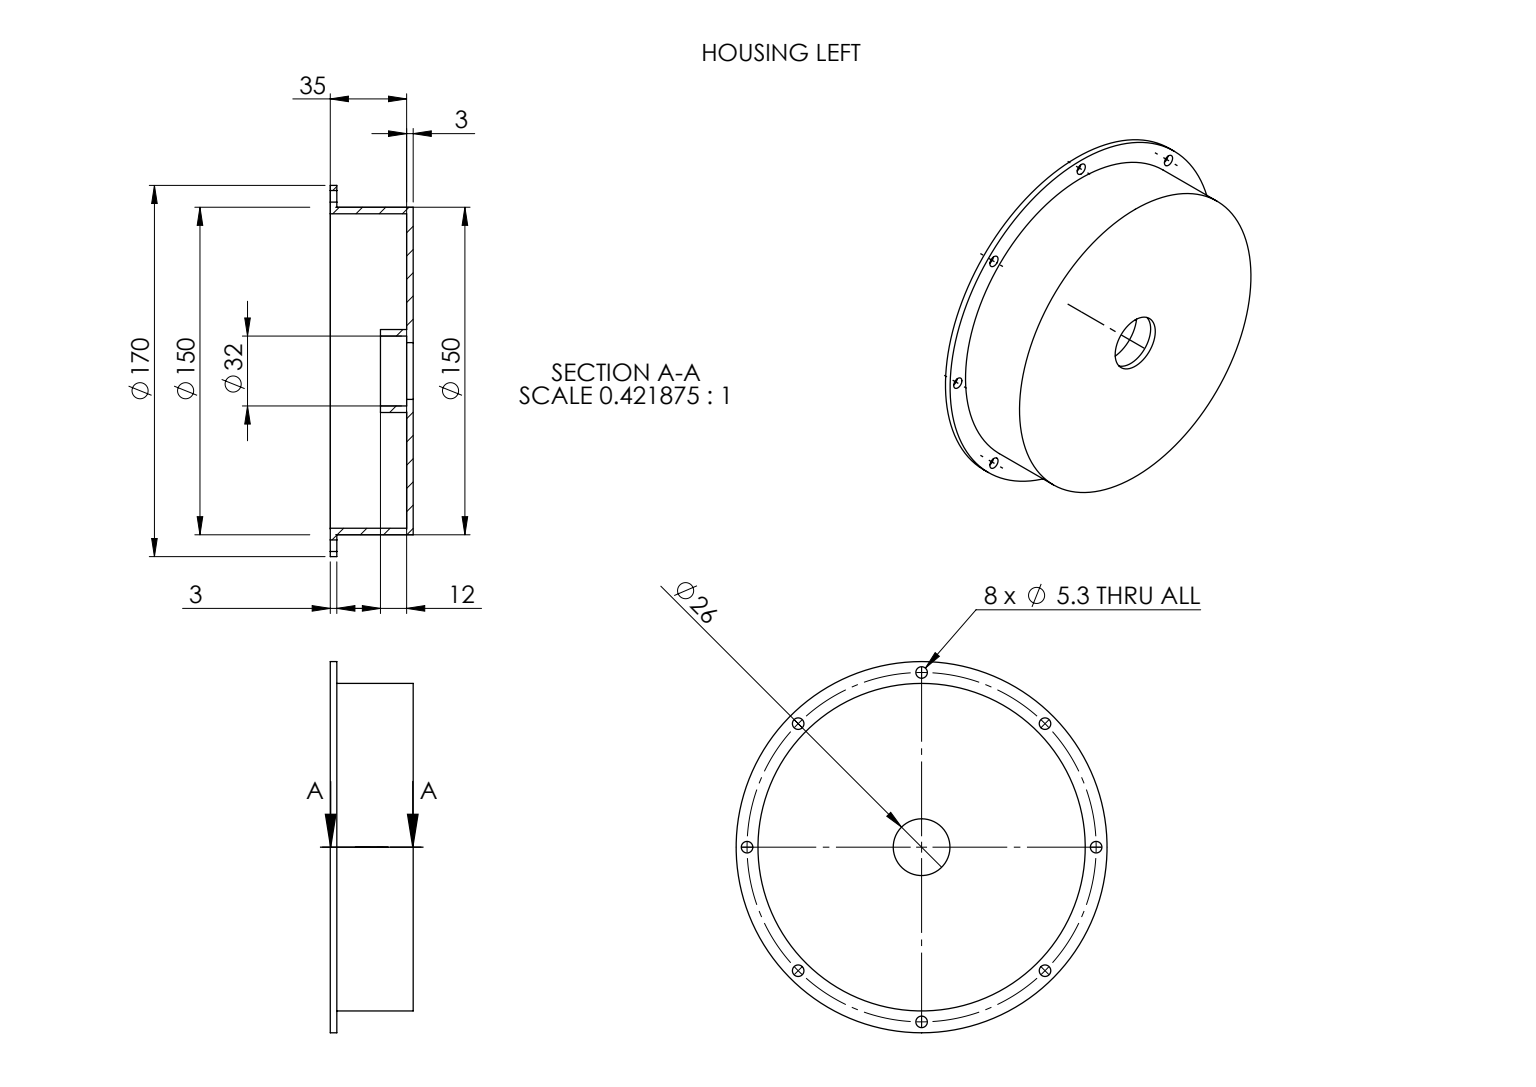
ISO-10303-21;
HEADER;
FILE_DESCRIPTION (('STEP AP214'),
    '1' );
FILE_NAME ('housing left.step',
    '2026-10-08T08:02:49',
    ( '' ),
    ( '' ),
    'SwSTEP 2.0',
    'SolidWorks 2026',
    '' );
FILE_SCHEMA (( 'AUTOMOTIVE_DESIGN' ));
ENDSEC;

DATA;
#22=CIRCLE ( 'NONE', #14059, 18.99999999999999645 ) ;
#26=ORIENTED_EDGE ( 'NONE', *, *, #59034, .F. ) ;
#28=CARTESIAN_POINT ( 'NONE',  ( 9.999999999999994671, 54.69470952477936976, 58.44237546506825964 ) ) ;
#114=DIRECTION ( 'NONE',  ( 0.000000000000000000, 0.7071067811865540120, -0.7071067811865409114 ) ) ;
#229=DIRECTION ( 'NONE',  ( -1.558861125776144859E-16, 1.000000000000000000, 0.000000000000000000 ) ) ;
#516=VERTEX_POINT ( 'NONE', #28669 ) ;
#583=FILL_AREA_STYLE_COLOUR ( '', #10848 ) ;
#732=EDGE_CURVE ( 'NONE', #32675, #50174, #22, .T. ) ;
#739=EDGE_LOOP ( 'NONE', ( #30578, #30226 ) ) ;
#851=EDGE_CURVE ( 'NONE', #38431, #10608, #42121, .T. ) ;
#979=CARTESIAN_POINT ( 'NONE',  ( 7.000000000000016875, -56.56854249492410958, 56.56854249492351983 ) ) ;
#1004=DIRECTION ( 'NONE',  ( 0.000000000000000000, 0.7071067811865500152, -0.7071067811865449082 ) ) ;
#1045=EDGE_CURVE ( 'NONE', #44352, #37554, #11099, .T. ) ;
#1056=AXIS2_PLACEMENT_3D ( 'NONE', #46617, #46933, #37219 ) ;
#1220=EDGE_LOOP ( 'NONE', ( #16192, #58248 ) ) ;
#1238=FACE_OUTER_BOUND ( 'NONE', #25127, .T. ) ;
#1308=ADVANCED_FACE ( 'NONE', ( #34786, #1238 ), #48554, .F. ) ;
#1325=EDGE_CURVE ( 'NONE', #18038, #2711, #15080, .T. ) ;
#1357=VERTEX_POINT ( 'NONE', #29143 ) ;
#1407=MECHANICAL_DESIGN_GEOMETRIC_PRESENTATION_REPRESENTATION('',(#54392),#17442);
#1450=EDGE_CURVE ( 'NONE', #1988, #10608, #40149, .T. ) ;
#1480=ORIENTED_EDGE ( 'NONE', *, *, #24999, .F. ) ;
#1544=ORIENTED_EDGE ( 'NONE', *, *, #24999, .T. ) ;
#1597=PRODUCT_DEFINITION_CONTEXT ( 'detailed design', #21992, 'design' ) ;
#1693=EDGE_LOOP ( 'NONE', ( #9790, #42814, #6756, #22247 ) ) ;
#1722=LINE ( 'NONE', #34653, #61604 ) ;
#1747=FACE_BOUND ( 'NONE', #39086, .T. ) ;
#1845=ORIENTED_EDGE ( 'NONE', *, *, #29444, .T. ) ;
#1874=VERTEX_POINT ( 'NONE', #54743 ) ;
#1982=VECTOR ( 'NONE', #50943, 1000.000000000000000 ) ;
#1983=FACE_BOUND ( 'NONE', #59580, .T. ) ;
#1988=VERTEX_POINT ( 'NONE', #18412 ) ;
#2034=ADVANCED_FACE ( 'NONE', ( #24026, #4272 ), #4895, .F. ) ;
#2113=DIRECTION ( 'NONE',  ( -1.000000000000000000, -1.836909530733573776E-16, 1.925929944387235853E-32 ) ) ;
#2157=EDGE_CURVE ( 'NONE', #55402, #25319, #24135, .T. ) ;
#2440=AXIS2_PLACEMENT_3D ( 'NONE', #41505, #59968, #8898 ) ;
#2557=DIRECTION ( 'NONE',  ( 0.000000000000000000, -1.000000000000000000, 0.000000000000000000 ) ) ;
#2571=CARTESIAN_POINT ( 'NONE',  ( 7.000000000000006217, 8.392413579938656024E-13, -80.00000000000001421 ) ) ;
#2625=EDGE_LOOP ( 'NONE', ( #36396, #26501, #31258, #19273 ) ) ;
#2659=AXIS2_PLACEMENT_3D ( 'NONE', #51775, #8874, #36245 ) ;
#2684=DIRECTION ( 'NONE',  ( -1.000000000000000000, -0.000000000000000000, -0.000000000000000000 ) ) ;
#2711=VERTEX_POINT ( 'NONE', #24485 ) ;
#2720=CIRCLE ( 'NONE', #37781, 2.649999999999999467 ) ;
#2736=ORIENTED_EDGE ( 'NONE', *, *, #34296, .T. ) ;
#2739=LINE ( 'NONE', #12480, #41873 ) ;
#2753=CIRCLE ( 'NONE', #37812, 2.649999999999985700 ) ;
#2770=CYLINDRICAL_SURFACE ( 'NONE', #48946, 2.649999999999992806 ) ;
#2778=DIRECTION ( 'NONE',  ( -1.000000000000000000, -1.836909530733573776E-16, 1.103352205049209901E-32 ) ) ;
#2817=MECHANICAL_DESIGN_GEOMETRIC_PRESENTATION_REPRESENTATION('',(#48840),#50847);
#2821=EDGE_CURVE ( 'NONE', #57549, #39665, #59140, .T. ) ;
#2917=EDGE_CURVE ( 'NONE', #47400, #1357, #48167, .T. ) ;
#3017=VERTEX_POINT ( 'NONE', #18490 ) ;
#3042=CARTESIAN_POINT ( 'NONE',  ( 42.00000000000000711, 6.547216728259810428E-15, -1.617781153285278467E-30 ) ) ;
#3179=EDGE_LOOP ( 'NONE', ( #47636, #54086, #41638, #28463 ) ) ;
#3190=CARTESIAN_POINT ( 'NONE',  ( 10.00000000000000533, 8.397924308530857731E-13, -80.00000000000001421 ) ) ;
#3221=DIRECTION ( 'NONE',  ( -1.000000000000000000, -0.000000000000000000, -0.000000000000000000 ) ) ;
#3238=ORIENTED_EDGE ( 'NONE', *, *, #53930, .F. ) ;
#3304=CARTESIAN_POINT ( 'NONE',  ( 42.00000000000000711, 7.715020029081011437E-15, -8.088905766426392334E-31 ) ) ;
#3387=VERTEX_POINT ( 'NONE', #31748 ) ;
#3408=ADVANCED_FACE ( 'NONE', ( #35844, #26731, #45253, #16411, #44942, #55220, #12654, #54282, #1983, #21108 ), #11405, .T. ) ;
#3479=VERTEX_POINT ( 'NONE', #8534 ) ;
#3488=DIRECTION ( 'NONE',  ( 1.000000000000000000, 1.836909530733573776E-16, -1.925929944387235579E-32 ) ) ;
#3501=DIRECTION ( 'NONE',  ( -1.000000000000000000, -5.380183451256670742E-17, 1.298891185607911324E-16 ) ) ;
#3546=CIRCLE ( 'NONE', #38604, 72.00000000000002842 ) ;
#3620=CARTESIAN_POINT ( 'NONE',  ( 7.000000000000016875, -54.69470952477895054, -58.44237546506863623 ) ) ;
#3624=CARTESIAN_POINT ( 'NONE',  ( 30.00000000000000711, 19.00000000000000000, -1.386669559958810165E-30 ) ) ;
#3759=CARTESIAN_POINT ( 'NONE',  ( 0.000000000000000000, 0.000000000000000000, 0.000000000000000000 ) ) ;
#3767=VECTOR ( 'NONE', #5831, 1000.000000000000000 ) ;
#3775=PRODUCT ( 'housing left', 'housing left', '', ( #26178 ) ) ;
#3842=DIRECTION ( 'NONE',  ( -1.000000000000000000, -3.135800716341471541E-16, -1.298891185607920445E-16 ) ) ;
#3848=CARTESIAN_POINT ( 'NONE',  ( 30.00000000000001066, 4.342925291379521108E-15, -1.386669559958810165E-30 ) ) ;
#3874=CARTESIAN_POINT ( 'NONE',  ( 7.000000000000021316, -80.00000000000001421, 2.649999999999992806 ) ) ;
#4007=VERTEX_POINT ( 'NONE', #26972 ) ;
#4020=EDGE_CURVE ( 'NONE', #3387, #24101, #40936, .T. ) ;
#4024=EDGE_LOOP ( 'NONE', ( #28100, #44874 ) ) ;
#4063=ORIENTED_EDGE ( 'NONE', *, *, #5152, .T. ) ;
#4173=DIRECTION ( 'NONE',  ( -1.000000000000000000, -1.836909530733573776E-16, 1.925929944387234758E-32 ) ) ;
#4221=ADVANCED_FACE ( 'NONE', ( #22092 ), #31172, .F. ) ;
#4236=EDGE_LOOP ( 'NONE', ( #11283, #12412 ) ) ;
#4258=CARTESIAN_POINT ( 'NONE',  ( 10.00000000000000533, 2.650000000000832134, -79.99999999999998579 ) ) ;
#4272=FACE_OUTER_BOUND ( 'NONE', #21523, .T. ) ;
#4292=DIRECTION ( 'NONE',  ( -1.826024711554534160E-16, 1.000000000000000000, 0.000000000000000000 ) ) ;
#4309=EDGE_CURVE ( 'NONE', #25319, #44352, #60010, .T. ) ;
#4456=AXIS2_PLACEMENT_3D ( 'NONE', #52364, #46164, #18264 ) ;
#4472=AXIS2_PLACEMENT_3D ( 'NONE', #56348, #47281, #33193 ) ;
#4491=CYLINDRICAL_SURFACE ( 'NONE', #43043, 15.99999999999999645 ) ;
#4503=CARTESIAN_POINT ( 'NONE',  ( 10.00000000000000888, -2.549224068967256091E-30, 75.00000000000001421 ) ) ;
#4529=AXIS2_PLACEMENT_3D ( 'NONE', #47141, #35361, #8584 ) ;
#4613=ORIENTED_EDGE ( 'NONE', *, *, #10966, .T. ) ;
#4647=ORIENTED_EDGE ( 'NONE', *, *, #16498, .T. ) ;
#4759=DIRECTION ( 'NONE',  ( -1.000000000000000000, -3.673819061467147552E-16, 1.925929944387234758E-32 ) ) ;
#4811=DIRECTION ( 'NONE',  ( -1.000000000000000000, -3.135800716341471541E-16, -1.298891185607920445E-16 ) ) ;
#4817=DIRECTION ( 'NONE',  ( 0.000000000000000000, 0.000000000000000000, 1.000000000000000000 ) ) ;
#4831=ADVANCED_BREP_SHAPE_REPRESENTATION ( '', ( #52245, #14677 ), #24835 ) ;
#4895=PLANE ( 'NONE',  #1056 ) ;
#4898=DIRECTION ( 'NONE',  ( 3.273063162220391312E-16, -1.000000000000000000, -5.236901059552626099E-15 ) ) ;
#4917=ORIENTED_EDGE ( 'NONE', *, *, #7261, .F. ) ;
#5152=EDGE_CURVE ( 'NONE', #20064, #24696, #61930, .T. ) ;
#5167=ORIENTED_EDGE ( 'NONE', *, *, #2821, .F. ) ;
#5171=LINE ( 'NONE', #6084, #41199 ) ;
#5227=ADVANCED_FACE ( 'NONE', ( #32227 ), #2770, .F. ) ;
#5259=EDGE_LOOP ( 'NONE', ( #10232, #39171, #52640, #43675 ) ) ;
#5271=CARTESIAN_POINT ( 'NONE',  ( 6.999999999999995559, 58.44237546506807490, 54.69470952477956871 ) ) ;
#5291=DIRECTION ( 'NONE',  ( -1.000000000000000000, -5.380183451256670742E-17, 1.298891185607911324E-16 ) ) ;
#5452=ORIENTED_EDGE ( 'NONE', *, *, #1325, .T. ) ;
#5519=FACE_BOUND ( 'NONE', #54215, .T. ) ;
#5603=ORIENTED_EDGE ( 'NONE', *, *, #43200, .F. ) ;
#5607=DIRECTION ( 'NONE',  ( -1.000000000000000000, -3.135800716341489291E-16, 1.298891185607901956E-16 ) ) ;
#5609=ORIENTED_EDGE ( 'NONE', *, *, #29444, .F. ) ;
#5821=DIRECTION ( 'NONE',  ( 1.836909530733573776E-16, -1.000000000000000000, 0.000000000000000000 ) ) ;
#5831=DIRECTION ( 'NONE',  ( -1.000000000000000000, -0.000000000000000000, -0.000000000000000000 ) ) ;
#5915=EDGE_LOOP ( 'NONE', ( #46556, #34430, #13398, #58645 ) ) ;
#6084=CARTESIAN_POINT ( 'NONE',  ( 6.999999999999992895, 72.00000000000002842, -1.348150961071066192E-31 ) ) ;
#6112=CARTESIAN_POINT ( 'NONE',  ( 30.00000000000000711, 16.00000000000000000, -1.502225356622044316E-30 ) ) ;
#6135=AXIS2_PLACEMENT_3D ( 'NONE', #35539, #54601, #49302 ) ;
#6151=CARTESIAN_POINT ( 'NONE',  ( 6.999999999999995559, 56.56854249492450037, -56.56854249492312192 ) ) ;
#6161=EDGE_CURVE ( 'NONE', #33929, #20064, #41040, .T. ) ;
#6225=DIRECTION ( 'NONE',  ( -1.000000000000000000, -3.135800716341471541E-16, -1.298891185607920445E-16 ) ) ;
#6490=VECTOR ( 'NONE', #52929, 1000.000000000000000 ) ;
#6576=CARTESIAN_POINT ( 'NONE',  ( 10.00000000000001599, -56.56854249492331377, -56.56854249492430142 ) ) ;
#6600=ORIENTED_EDGE ( 'NONE', *, *, #12325, .T. ) ;
#6625=DIRECTION ( 'NONE',  ( -3.273063162220391312E-16, 1.000000000000000000, 1.047380211910525220E-14 ) ) ;
#6709=DIRECTION ( 'NONE',  ( 1.836766033387207149E-16, -1.000000000000000000, 0.000000000000000000 ) ) ;
#6756=ORIENTED_EDGE ( 'NONE', *, *, #44992, .T. ) ;
#6760=SHAPE_REPRESENTATION ( 'housing left', ( #14677 ), #24835 ) ;
#6863=AXIS2_PLACEMENT_3D ( 'NONE', #23333, #47761, #37770 ) ;
#7077=CARTESIAN_POINT ( 'NONE',  ( 42.00000000000000711, 1.592040838891559293E-15, -13.00000000000000178 ) ) ;
#7123=FACE_BOUND ( 'NONE', #19230, .T. ) ;
#7125=CIRCLE ( 'NONE', #18162, 2.649999999999997691 ) ;
#7151=LINE ( 'NONE', #12514, #53981 ) ;
#7225=CARTESIAN_POINT ( 'NONE',  ( 45.00000000000001421, 0.000000000000000000, 0.000000000000000000 ) ) ;
#7261=EDGE_CURVE ( 'NONE', #50174, #32675, #28553, .T. ) ;
#7264=CARTESIAN_POINT ( 'NONE',  ( 9.999999999999991118, 80.00000000000001421, 2.649999999999992806 ) ) ;
#7288=CARTESIAN_POINT ( 'NONE',  ( 7.000000000000006217, 1.285836671513502038E-15, -1.348150961071066192E-31 ) ) ;
#7300=CYLINDRICAL_SURFACE ( 'NONE', #35562, 18.99999999999999645 ) ;
#7334=EDGE_CURVE ( 'NONE', #43245, #53393, #46557, .T. ) ;
#7452=ORIENTED_EDGE ( 'NONE', *, *, #34318, .F. ) ;
#7487=EDGE_LOOP ( 'NONE', ( #36785, #12533, #57073, #23756 ) ) ;
#7625=DIRECTION ( 'NONE',  ( 0.000000000000000000, 0.000000000000000000, 1.000000000000000000 ) ) ;
#7658=VECTOR ( 'NONE', #27391, 1000.000000000000000 ) ;
#7679=EDGE_LOOP ( 'NONE', ( #1480, #38792, #47540, #22144 ) ) ;
#7754=DIRECTION ( 'NONE',  ( -1.000000000000000000, -1.836909530733573776E-16, 1.925929944387235853E-32 ) ) ;
#7877=PRODUCT_DEFINITION_FORMATION_WITH_SPECIFIED_SOURCE ( 'ANY', '', #3775, .NOT_KNOWN. ) ;
#7972=LINE ( 'NONE', #3874, #59630 ) ;
#7976=FACE_OUTER_BOUND ( 'NONE', #29688, .T. ) ;
#8009=DIRECTION ( 'NONE',  ( 0.000000000000000000, -1.047444401652941269E-14, 1.000000000000000000 ) ) ;
#8045=DIRECTION ( 'NONE',  ( -1.000000000000000000, -5.380183451256491399E-17, -1.298891185607892835E-16 ) ) ;
#8080=DIRECTION ( 'NONE',  ( -1.000000000000000000, -1.836909530733573776E-16, 1.925929944387235853E-32 ) ) ;
#8132=CYLINDRICAL_SURFACE ( 'NONE', #55782, 2.649999999999992806 ) ;
#8262=CARTESIAN_POINT ( 'NONE',  ( 10.00000000000002132, -80.00000000000001421, -2.532597876869216023E-31 ) ) ;
#8320=EDGE_CURVE ( 'NONE', #31692, #49531, #27575, .T. ) ;
#8342=EDGE_CURVE ( 'NONE', #37554, #44352, #15472, .T. ) ;
#8380=CARTESIAN_POINT ( 'NONE',  ( 9.999999999999994671, 56.56854249492371878, 56.56854249492391062 ) ) ;
#8397=EDGE_CURVE ( 'NONE', #27868, #516, #34480, .T. ) ;
#8400=ORIENTED_EDGE ( 'NONE', *, *, #16729, .F. ) ;
#8401=DIRECTION ( 'NONE',  ( 0.000000000000000000, 0.7071067811865500152, -0.7071067811865449082 ) ) ;
#8534=CARTESIAN_POINT ( 'NONE',  ( 7.000000000000005329, 2.649999999999721467, 80.00000000000002842 ) ) ;
#8584=DIRECTION ( 'NONE',  ( 0.000000000000000000, -1.000000000000000000, 0.000000000000000000 ) ) ;
#8603=DIRECTION ( 'NONE',  ( -1.000000000000000000, -0.000000000000000000, 1.925929944387235853E-32 ) ) ;
#8789=DIRECTION ( 'NONE',  ( -1.000000000000000000, -1.836909530733573529E-16, 1.361838123766461297E-32 ) ) ;
#8842=AXIS2_PLACEMENT_3D ( 'NONE', #54750, #8080, #13112 ) ;
#8874=DIRECTION ( 'NONE',  ( 1.000000000000000000, 1.836909530733573776E-16, -1.925929944387235853E-32 ) ) ;
#8883=EDGE_LOOP ( 'NONE', ( #35923, #47412 ) ) ;
#8888=ORIENTED_EDGE ( 'NONE', *, *, #56001, .F. ) ;
#8898=DIRECTION ( 'NONE',  ( 0.000000000000000000, 0.000000000000000000, 1.000000000000000000 ) ) ;
#8973=EDGE_CURVE ( 'NONE', #49007, #4007, #56449, .T. ) ;
#9009=EDGE_CURVE ( 'NONE', #38620, #38431, #11443, .T. ) ;
#9123=EDGE_LOOP ( 'NONE', ( #47938, #5609 ) ) ;
#9159=ORIENTED_EDGE ( 'NONE', *, *, #8320, .F. ) ;
#9166=EDGE_LOOP ( 'NONE', ( #13444, #4647 ) ) ;
#9171=CARTESIAN_POINT ( 'NONE',  ( 7.000000000000016875, -58.44237546506767700, -54.69470952477997372 ) ) ;
#9411=VECTOR ( 'NONE', #61831, 1000.000000000000000 ) ;
#9526=DIRECTION ( 'NONE',  ( 0.000000000000000000, -0.7071067811865487940, 0.7071067811865461294 ) ) ;
#9630=CARTESIAN_POINT ( 'NONE',  ( 7.000000000000021316, -80.00000000000001421, -1.954818893553044610E-31 ) ) ;
#9659=CARTESIAN_POINT ( 'NONE',  ( 7.000000000000016875, -54.69470952477976056, 58.44237546506787595 ) ) ;
#9693=CIRCLE ( 'NONE', #17708, 2.649999999999992806 ) ;
#9709=ADVANCED_FACE ( 'NONE', ( #18164 ), #48208, .F. ) ;
#9788=UNCERTAINTY_MEASURE_WITH_UNIT (LENGTH_MEASURE( 1.000000000000000082E-05 ), #33208, 'distance_accuracy_value', 'NONE');
#9790=ORIENTED_EDGE ( 'NONE', *, *, #22745, .F. ) ;
#9827=VECTOR ( 'NONE', #60704, 1000.000000000000000 ) ;
#9845=CARTESIAN_POINT ( 'NONE',  ( 9.999999999999994671, 56.56854249492450037, -56.56854249492312192 ) ) ;
#9868=AXIS2_PLACEMENT_3D ( 'NONE', #18102, #56295, #4898 ) ;
#9935=CARTESIAN_POINT ( 'NONE',  ( 10.00000000000000533, -2.774815975767171530E-13, 80.00000000000001421 ) ) ;
#9946=AXIS2_PLACEMENT_3D ( 'NONE', #56969, #14091, #23465 ) ;
#9955=VERTEX_POINT ( 'NONE', #4258 ) ;
#9981=ORIENTED_EDGE ( 'NONE', *, *, #53884, .F. ) ;
#10001=DIRECTION ( 'NONE',  ( -1.000000000000000000, -1.836909530733573776E-16, 1.925929944387235853E-32 ) ) ;
#10024=AXIS2_PLACEMENT_3D ( 'NONE', #54408, #20618, #21538 ) ;
#10169=LINE ( 'NONE', #15186, #22435 ) ;
#10170=CARTESIAN_POINT ( 'NONE',  ( 30.00000000000000711, 19.00000000000000000, -1.502225356622044491E-30 ) ) ;
#10232=ORIENTED_EDGE ( 'NONE', *, *, #4309, .F. ) ;
#10305=CARTESIAN_POINT ( 'NONE',  ( 42.00000000000000711, 7.715020029081011437E-15, -8.088905766426392334E-31 ) ) ;
#10352=CYLINDRICAL_SURFACE ( 'NONE', #55342, 2.649999999999992806 ) ;
#10557=CARTESIAN_POINT ( 'NONE',  ( 10.00000000000000533, 1.836909530733574959E-15, -1.925929944387237167E-31 ) ) ;
#10560=AXIS2_PLACEMENT_3D ( 'NONE', #40517, #17934, #45518 ) ;
#10571=LINE ( 'NONE', #43487, #3767 ) ;
#10600=AXIS2_PLACEMENT_3D ( 'NONE', #21436, #25823, #44051 ) ;
#10608=VERTEX_POINT ( 'NONE', #36068 ) ;
#10659=EDGE_LOOP ( 'NONE', ( #45292, #2736, #4613, #16201 ) ) ;
#10848=COLOUR_RGB ( '', 0.72549020, 0.75294118, 0.79215686) ;
#10882=VERTEX_POINT ( 'NONE', #41016 ) ;
#10966=EDGE_CURVE ( 'NONE', #3479, #38027, #40790, .T. ) ;
#10974=CIRCLE ( 'NONE', #9946, 15.99999999999999645 ) ;
#11058=ORIENTED_EDGE ( 'NONE', *, *, #8973, .F. ) ;
#11099=CIRCLE ( 'NONE', #26065, 13.00000000000000178 ) ;
#11176=EDGE_LOOP ( 'NONE', ( #35468, #31545 ) ) ;
#11178=FACE_BOUND ( 'NONE', #11176, .T. ) ;
#11283=ORIENTED_EDGE ( 'NONE', *, *, #59034, .T. ) ;
#11405=PLANE ( 'NONE',  #61848 ) ;
#11411=COLOUR_RGB ( '', 0.72549020, 0.75294118, 0.79215686) ;
#11443=CIRCLE ( 'NONE', #54432, 2.649999999999985700 ) ;
#11448=SURFACE_STYLE_FILL_AREA ( #54325 ) ;
#11558=( NAMED_UNIT ( * ) SI_UNIT ( $, .STERADIAN. ) SOLID_ANGLE_UNIT ( ) );
#11613=DIRECTION ( 'NONE',  ( -1.000000000000000000, -0.000000000000000000, 1.925929944387235853E-32 ) ) ;
#11754=DIRECTION ( 'NONE',  ( -1.000000000000000000, -1.836909530733573776E-16, 1.925929944387235853E-32 ) ) ;
#11785=ORIENTED_EDGE ( 'NONE', *, *, #50491, .F. ) ;
#11792=AXIS2_PLACEMENT_3D ( 'NONE', #10305, #10001, #43528 ) ;
#11823=DIRECTION ( 'NONE',  ( -1.000000000000000000, -1.836909530733554547E-16, -1.836909530733573529E-16 ) ) ;
#11882=( NAMED_UNIT ( * ) PLANE_ANGLE_UNIT ( ) SI_UNIT ( $, .RADIAN. ) );
#11884=ADVANCED_FACE ( 'NONE', ( #57840 ), #57519, .F. ) ;
#11918=DIRECTION ( 'NONE',  ( -3.273063162220391312E-16, 1.000000000000000000, 1.047380211910525220E-14 ) ) ;
#11927=VERTEX_POINT ( 'NONE', #42547 ) ;
#11937=DIRECTION ( 'NONE',  ( -1.000000000000000000, -1.836909530733573776E-16, 1.925929944387235579E-32 ) ) ;
#12013=DIRECTION ( 'NONE',  ( -1.000000000000000000, -1.836909530733554547E-16, -1.836909530733573529E-16 ) ) ;
#12057=CIRCLE ( 'NONE', #10024, 2.649999999999985700 ) ;
#12076=EDGE_CURVE ( 'NONE', #33012, #9955, #23763, .T. ) ;
#12106=CARTESIAN_POINT ( 'NONE',  ( 6.999999999999995559, 56.56854249492371878, 56.56854249492391062 ) ) ;
#12298=CARTESIAN_POINT ( 'NONE',  ( 10.00000000000000533, 1.836909530733574959E-15, -1.925929944387237167E-31 ) ) ;
#12325=EDGE_CURVE ( 'NONE', #55726, #516, #61534, .T. ) ;
#12354=UNCERTAINTY_MEASURE_WITH_UNIT (LENGTH_MEASURE( 1.000000000000000082E-05 ), #30532, 'distance_accuracy_value', 'NONE');
#12385=PRESENTATION_STYLE_ASSIGNMENT (( #12696 ) ) ;
#12412=ORIENTED_EDGE ( 'NONE', *, *, #27510, .T. ) ;
#12480=CARTESIAN_POINT ( 'NONE',  ( 7.000000000000016875, -54.69470952477976766, 58.44237546506786884 ) ) ;
#12514=CARTESIAN_POINT ( 'NONE',  ( 7.000000000000016875, -54.69470952477895764, -58.44237546506863623 ) ) ;
#12533=ORIENTED_EDGE ( 'NONE', *, *, #7334, .F. ) ;
#12572=DIRECTION ( 'NONE',  ( 0.000000000000000000, 0.7071067811865421326, 0.7071067811865527908 ) ) ;
#12633=AXIS2_PLACEMENT_3D ( 'NONE', #60676, #7754, #32203 ) ;
#12652=VERTEX_POINT ( 'NONE', #38017 ) ;
#12654=FACE_BOUND ( 'NONE', #9123, .T. ) ;
#12696=SURFACE_STYLE_USAGE ( .BOTH. , #55261 ) ;
#12744=CARTESIAN_POINT ( 'NONE',  ( 7.000000000000006217, -2.780326704359372228E-13, 80.00000000000001421 ) ) ;
#12862=CARTESIAN_POINT ( 'NONE',  ( 10.00000000000001599, -54.69470952477895764, -58.44237546506863623 ) ) ;
#12995=AXIS2_PLACEMENT_3D ( 'NONE', #9935, #52832, #33750 ) ;
#13092=EDGE_LOOP ( 'NONE', ( #36741, #22358 ) ) ;
#13094=DIRECTION ( 'NONE',  ( -1.000000000000000000, -3.135800716341489291E-16, 1.298891185607901956E-16 ) ) ;
#13112=DIRECTION ( 'NONE',  ( 1.836766033387207149E-16, -1.000000000000000000, 0.000000000000000000 ) ) ;
#13183=EDGE_CURVE ( 'NONE', #4007, #49007, #2720, .T. ) ;
#13215=DIRECTION ( 'NONE',  ( -1.000000000000000000, -1.836909530733573776E-16, 1.925929944387235853E-32 ) ) ;
#13335=EDGE_CURVE ( 'NONE', #37250, #55180, #1722, .T. ) ;
#13365=CARTESIAN_POINT ( 'NONE',  ( 6.999999999999991118, 80.00000000000001421, 2.649999999999992806 ) ) ;
#13370=AXIS2_PLACEMENT_3D ( 'NONE', #15636, #2113, #39767 ) ;
#13378=CARTESIAN_POINT ( 'NONE',  ( 7.000000000000021316, -80.00000000000001421, -1.954818893553044610E-31 ) ) ;
#13398=ORIENTED_EDGE ( 'NONE', *, *, #8342, .F. ) ;
#13428=CIRCLE ( 'NONE', #14460, 2.649999999999985700 ) ;
#13438=ORIENTED_EDGE ( 'NONE', *, *, #49569, .F. ) ;
#13444=ORIENTED_EDGE ( 'NONE', *, *, #15200, .T. ) ;
#13542=DIRECTION ( 'NONE',  ( -1.000000000000000000, -1.836909530733573776E-16, 2.465190328815682145E-32 ) ) ;
#13668=CYLINDRICAL_SURFACE ( 'NONE', #53195, 2.649999999999992806 ) ;
#13731=CARTESIAN_POINT ( 'NONE',  ( 42.00000000000002132, -72.00000000000001421, 8.817456953860944867E-15 ) ) ;
#13822=DIRECTION ( 'NONE',  ( 1.000000000000000000, 0.000000000000000000, 0.000000000000000000 ) ) ;
#13857=EDGE_LOOP ( 'NONE', ( #46722, #41790, #37267, #41170 ) ) ;
#13872=CIRCLE ( 'NONE', #19861, 2.649999999999997691 ) ;
#14026=AXIS2_PLACEMENT_3D ( 'NONE', #37146, #32432, #56216 ) ;
#14059=AXIS2_PLACEMENT_3D ( 'NONE', #59948, #17057, #7625 ) ;
#14091=DIRECTION ( 'NONE',  ( -1.000000000000000000, -1.836909530733573776E-16, 1.925929944387235853E-32 ) ) ;
#14269=LINE ( 'NONE', #42776, #9411 ) ;
#14408=PRESENTATION_STYLE_ASSIGNMENT (( #58209 ) ) ;
#14460=AXIS2_PLACEMENT_3D ( 'NONE', #3190, #13542, #32647 ) ;
#14517=ORIENTED_EDGE ( 'NONE', *, *, #8397, .T. ) ;
#14542=ORIENTED_EDGE ( 'NONE', *, *, #29380, .F. ) ;
#14547=ORIENTED_EDGE ( 'NONE', *, *, #23645, .T. ) ;
#14586=ORIENTED_EDGE ( 'NONE', *, *, #55140, .T. ) ;
#14677=AXIS2_PLACEMENT_3D ( 'NONE', #3759, #61387, #13822 ) ;
#14793=DIRECTION ( 'NONE',  ( -1.000000000000000000, -3.135800716341489291E-16, 1.298891185607901956E-16 ) ) ;
#14822=DIRECTION ( 'NONE',  ( 1.000000000000000000, 1.558861125776144859E-16, -3.851859888774471706E-32 ) ) ;
#14845=CARTESIAN_POINT ( 'NONE',  ( 6.999999999999995559, 58.44237546506882808, -54.69470952477875159 ) ) ;
#14904=CIRCLE ( 'NONE', #50864, 75.00000000000001421 ) ;
#14968=DIRECTION ( 'NONE',  ( -2.168404344971009361E-16, 1.000000000000000000, 0.000000000000000000 ) ) ;
#14997=FACE_OUTER_BOUND ( 'NONE', #36041, .T. ) ;
#15011=ORIENTED_EDGE ( 'NONE', *, *, #60867, .F. ) ;
#15080=CIRCLE ( 'NONE', #43126, 72.00000000000002842 ) ;
#15112=EDGE_LOOP ( 'NONE', ( #47046, #8400, #30914, #19464 ) ) ;
#15117=ORIENTED_EDGE ( 'NONE', *, *, #9009, .T. ) ;
#15186=CARTESIAN_POINT ( 'NONE',  ( 7.000000000000005329, 2.649999999999714806, 80.00000000000002842 ) ) ;
#15200=EDGE_CURVE ( 'NONE', #18005, #35841, #7125, .T. ) ;
#15268=FACE_OUTER_BOUND ( 'NONE', #23044, .T. ) ;
#15429=ORIENTED_EDGE ( 'NONE', *, *, #32636, .T. ) ;
#15472=CIRCLE ( 'NONE', #39502, 13.00000000000000178 ) ;
#15571=AXIS2_PLACEMENT_3D ( 'NONE', #51698, #8789, #18508 ) ;
#15636=CARTESIAN_POINT ( 'NONE',  ( 10.00000000000000533, 1.836909530733574959E-15, -1.925929944387237167E-31 ) ) ;
#15641=ADVANCED_FACE ( 'NONE', ( #47472 ), #23660, .F. ) ;
#15682=CARTESIAN_POINT ( 'NONE',  ( 7.000000000000006217, 1.285836671513502038E-15, -1.348150961071066192E-31 ) ) ;
#15841=ORIENTED_EDGE ( 'NONE', *, *, #34296, .F. ) ;
#15980=VECTOR ( 'NONE', #46485, 1000.000000000000000 ) ;
#16024=AXIS2_PLACEMENT_3D ( 'NONE', #25240, #59665, #34972 ) ;
#16064=CIRCLE ( 'NONE', #17054, 2.649999999999997691 ) ;
#16073=ADVANCED_FACE ( 'NONE', ( #32225 ), #52226, .T. ) ;
#16082=ORIENTED_EDGE ( 'NONE', *, *, #15200, .F. ) ;
#16192=ORIENTED_EDGE ( 'NONE', *, *, #8342, .T. ) ;
#16201=ORIENTED_EDGE ( 'NONE', *, *, #59116, .F. ) ;
#16209=FACE_OUTER_BOUND ( 'NONE', #3179, .T. ) ;
#16287=CARTESIAN_POINT ( 'NONE',  ( 7.000000000000007105, -2.650000000000277467, 80.00000000000000000 ) ) ;
#16341=EDGE_LOOP ( 'NONE', ( #49112, #23294 ) ) ;
#16345=ADVANCED_FACE ( 'NONE', ( #37169 ), #13668, .F. ) ;
#16411=FACE_BOUND ( 'NONE', #49120, .T. ) ;
#16445=AXIS2_PLACEMENT_3D ( 'NONE', #12298, #21676, #59883 ) ;
#16451=( NAMED_UNIT ( * ) PLANE_ANGLE_UNIT ( ) SI_UNIT ( $, .RADIAN. ) );
#16498=EDGE_CURVE ( 'NONE', #35841, #18005, #48249, .T. ) ;
#16514=DIRECTION ( 'NONE',  ( 0.000000000000000000, 0.7071067811865395791, 0.7071067811865553443 ) ) ;
#16635=ADVANCED_FACE ( 'NONE', ( #42379 ), #56745, .F. ) ;
#16729=EDGE_CURVE ( 'NONE', #12652, #33929, #35291, .T. ) ;
#16825=CARTESIAN_POINT ( 'NONE',  ( 7.000000000000007105, -2.649999999999153477, -80.00000000000004263 ) ) ;
#16957=AXIS2_PLACEMENT_3D ( 'NONE', #49657, #55272, #17095 ) ;
#17054=AXIS2_PLACEMENT_3D ( 'NONE', #33982, #4811, #114 ) ;
#17057=DIRECTION ( 'NONE',  ( -1.000000000000000000, -1.836909530733573776E-16, 1.925929944387235853E-32 ) ) ;
#17092=VECTOR ( 'NONE', #4759, 1000.000000000000000 ) ;
#17095=DIRECTION ( 'NONE',  ( -3.273063162220399693E-16, 1.000000000000000000, 1.047380211910527902E-14 ) ) ;
#17222=AXIS2_PLACEMENT_3D ( 'NONE', #51302, #31913, #4292 ) ;
#17369=DIRECTION ( 'NONE',  ( 1.000000000000000000, 1.558861125776144859E-16, -3.851859888774471706E-32 ) ) ;
#17442=( GEOMETRIC_REPRESENTATION_CONTEXT ( 3 ) GLOBAL_UNCERTAINTY_ASSIGNED_CONTEXT ( ( #12354 ) ) GLOBAL_UNIT_ASSIGNED_CONTEXT ( ( #30532, #16451, #50570 ) ) REPRESENTATION_CONTEXT ( 'NONE', 'WORKASPACE' ) );
#17465=DIRECTION ( 'NONE',  ( 0.000000000000000000, 1.000000000000000000, 0.000000000000000000 ) ) ;
#17509=ORIENTED_EDGE ( 'NONE', *, *, #30916, .T. ) ;
#17573=EDGE_LOOP ( 'NONE', ( #5452, #14586, #52896, #41125 ) ) ;
#17630=CARTESIAN_POINT ( 'NONE',  ( 9.999999999999994671, 56.56854249492371878, 56.56854249492391062 ) ) ;
#17683=DIRECTION ( 'NONE',  ( -1.000000000000000000, -3.135800716341471541E-16, -1.298891185607920445E-16 ) ) ;
#17702=DIRECTION ( 'NONE',  ( -1.000000000000000000, -3.673819061467147552E-16, 1.925929944387234758E-32 ) ) ;
#17708=AXIS2_PLACEMENT_3D ( 'NONE', #59654, #59035, #44369 ) ;
#17754=EDGE_LOOP ( 'NONE', ( #5167, #59322 ) ) ;
#17784=DIRECTION ( 'NONE',  ( 0.000000000000000000, -0.7071067811865435759, -0.7071067811865514585 ) ) ;
#17812=CARTESIAN_POINT ( 'NONE',  ( 7.000000000000006217, 1.285836671513502038E-15, -1.348150961071066192E-31 ) ) ;
#17828=CARTESIAN_POINT ( 'NONE',  ( 10.00000000000001599, -56.56854249492410958, 56.56854249492351983 ) ) ;
#17934=DIRECTION ( 'NONE',  ( -1.000000000000000000, -1.836909530733573776E-16, 1.925929944387235853E-32 ) ) ;
#18005=VERTEX_POINT ( 'NONE', #28 ) ;
#18038=VERTEX_POINT ( 'NONE', #24466 ) ;
#18051=ORIENTED_EDGE ( 'NONE', *, *, #2157, .F. ) ;
#18102=CARTESIAN_POINT ( 'NONE',  ( 7.000000000000006217, -2.780326704359372228E-13, 80.00000000000001421 ) ) ;
#18162=AXIS2_PLACEMENT_3D ( 'NONE', #8380, #56923, #27500 ) ;
#18164=FACE_OUTER_BOUND ( 'NONE', #5259, .T. ) ;
#18244=CARTESIAN_POINT ( 'NONE',  ( 9.999999999999994671, 58.44237546506882808, -54.69470952477875869 ) ) ;
#18264=DIRECTION ( 'NONE',  ( 0.000000000000000000, 3.491481338843138088E-15, -1.000000000000000000 ) ) ;
#18348=CARTESIAN_POINT ( 'NONE',  ( 6.999999999999991118, 80.00000000000001421, -7.414830285890871171E-32 ) ) ;
#18351=ORIENTED_EDGE ( 'NONE', *, *, #26090, .T. ) ;
#18379=EDGE_LOOP ( 'NONE', ( #32883, #4917, #59902, #18351 ) ) ;
#18393=EDGE_CURVE ( 'NONE', #45374, #21079, #45827, .T. ) ;
#18412=CARTESIAN_POINT ( 'NONE',  ( 7.000000000000021316, -80.00000000000001421, 2.649999999999999467 ) ) ;
#18490=CARTESIAN_POINT ( 'NONE',  ( 7.000000000000022204, -85.00000000000001421, -1.348150961071066192E-31 ) ) ;
#18508=DIRECTION ( 'NONE',  ( 0.000000000000000000, -0.7071067811865553443, 0.7071067811865395791 ) ) ;
#18520=VECTOR ( 'NONE', #45969, 1000.000000000000000 ) ;
#18659=ORIENTED_EDGE ( 'NONE', *, *, #59898, .T. ) ;
#18763=CARTESIAN_POINT ( 'NONE',  ( 6.999999999999995559, 54.69470952478017267, -58.44237546506749936 ) ) ;
#18914=DIRECTION ( 'NONE',  ( 0.000000000000000000, 0.000000000000000000, 1.000000000000000000 ) ) ;
#18942=EDGE_LOOP ( 'NONE', ( #15841, #27522, #35878, #14547 ) ) ;
#18950=FACE_OUTER_BOUND ( 'NONE', #36016, .T. ) ;
#19114=SURFACE_SIDE_STYLE ('',( #57274 ) ) ;
#19230=EDGE_LOOP ( 'NONE', ( #55552, #29522 ) ) ;
#19273=ORIENTED_EDGE ( 'NONE', *, *, #59634, .F. ) ;
#19328=CARTESIAN_POINT ( 'NONE',  ( 10.00000000000000533, 1.836909530733574959E-15, -1.925929944387237167E-31 ) ) ;
#19369=ORIENTED_EDGE ( 'NONE', *, *, #18393, .T. ) ;
#19380=FACE_BOUND ( 'NONE', #53090, .T. ) ;
#19401=EDGE_LOOP ( 'NONE', ( #24342, #48250 ) ) ;
#19464=ORIENTED_EDGE ( 'NONE', *, *, #5152, .F. ) ;
#19632=ORIENTED_EDGE ( 'NONE', *, *, #36032, .T. ) ;
#19691=ORIENTED_EDGE ( 'NONE', *, *, #32636, .F. ) ;
#19717=FILL_AREA_STYLE ('',( #583 ) ) ;
#19861=AXIS2_PLACEMENT_3D ( 'NONE', #25866, #59991, #49986 ) ;
#19995=ORIENTED_EDGE ( 'NONE', *, *, #1325, .F. ) ;
#20064=VERTEX_POINT ( 'NONE', #56607 ) ;
#20223=ORIENTED_EDGE ( 'NONE', *, *, #36242, .T. ) ;
#20270=CARTESIAN_POINT ( 'NONE',  ( 45.00000000000001421, 9.184850993605151889E-15, -75.00000000000001421 ) ) ;
#20346=APPLICATION_CONTEXT ( 'automotive_design' ) ;
#20348=ADVANCED_FACE ( 'NONE', ( #55912 ), #32131, .F. ) ;
#20358=AXIS2_PLACEMENT_3D ( 'NONE', #39813, #6225, #25675 ) ;
#20392=ORIENTED_EDGE ( 'NONE', *, *, #12076, .T. ) ;
#20464=CARTESIAN_POINT ( 'NONE',  ( 45.00000000000001421, 0.000000000000000000, 0.000000000000000000 ) ) ;
#20575=CIRCLE ( 'NONE', #10560, 15.99999999999999645 ) ;
#20582=FACE_OUTER_BOUND ( 'NONE', #29977, .T. ) ;
#20613=CIRCLE ( 'NONE', #10600, 2.649999999999985700 ) ;
#20618=DIRECTION ( 'NONE',  ( -1.000000000000000000, -1.836909530733573776E-16, 1.925929944387235853E-32 ) ) ;
#20679=DIRECTION ( 'NONE',  ( 0.000000000000000000, -0.7071067811865449082, -0.7071067811865500152 ) ) ;
#20722=EDGE_CURVE ( 'NONE', #27605, #47270, #31450, .T. ) ;
#20762=ORIENTED_EDGE ( 'NONE', *, *, #38598, .T. ) ;
#20933=AXIS2_PLACEMENT_3D ( 'NONE', #59427, #25933, #45070 ) ;
#20955=DIRECTION ( 'NONE',  ( 0.000000000000000000, 0.000000000000000000, -1.000000000000000000 ) ) ;
#20982=CARTESIAN_POINT ( 'NONE',  ( 7.000000000000006217, 8.392413579938656024E-13, -80.00000000000001421 ) ) ;
#20998=CARTESIAN_POINT ( 'NONE',  ( 9.999999999999991118, 80.00000000000001421, -1.319262011905257654E-31 ) ) ;
#21079=VERTEX_POINT ( 'NONE', #13731 ) ;
#21108=FACE_OUTER_BOUND ( 'NONE', #4024, .T. ) ;
#21436=CARTESIAN_POINT ( 'NONE',  ( 10.00000000000002132, -80.00000000000001421, -2.532597876869216023E-31 ) ) ;
#21460=CARTESIAN_POINT ( 'NONE',  ( 10.00000000000000533, 1.836909530733574959E-15, -1.925929944387237167E-31 ) ) ;
#21495=EDGE_LOOP ( 'NONE', ( #15429, #46374, #13438, #52011 ) ) ;
#21518=DIRECTION ( 'NONE',  ( -1.000000000000000000, -5.380183451256491399E-17, -1.298891185607892835E-16 ) ) ;
#21523=EDGE_LOOP ( 'NONE', ( #14517, #33977 ) ) ;
#21538=DIRECTION ( 'NONE',  ( 0.000000000000000000, -1.000000000000000000, 0.000000000000000000 ) ) ;
#21586=DIRECTION ( 'NONE',  ( -1.000000000000000000, -5.380183451256491399E-17, -1.298891185607892835E-16 ) ) ;
#21642=AXIS2_PLACEMENT_3D ( 'NONE', #50953, #8045, #36890 ) ;
#21676=DIRECTION ( 'NONE',  ( -1.000000000000000000, -1.836909530733573776E-16, 1.925929944387235853E-32 ) ) ;
#21690=CARTESIAN_POINT ( 'NONE',  ( 7.000000000000005329, 2.650000000000831690, -79.99999999999998579 ) ) ;
#21700=EDGE_CURVE ( 'NONE', #55402, #37554, #55226, .T. ) ;
#21739=LINE ( 'NONE', #59944, #15980 ) ;
#21794=CYLINDRICAL_SURFACE ( 'NONE', #47994, 2.649999999999997691 ) ;
#21826=DIRECTION ( 'NONE',  ( -1.000000000000000000, -3.135800716341489291E-16, 1.298891185607901956E-16 ) ) ;
#21827=ORIENTED_EDGE ( 'NONE', *, *, #47810, .T. ) ;
#21906=AXIS2_PLACEMENT_3D ( 'NONE', #28811, #5291, #24418 ) ;
#21927=ORIENTED_EDGE ( 'NONE', *, *, #40080, .T. ) ;
#21933=EDGE_CURVE ( 'NONE', #25319, #55402, #34702, .T. ) ;
#21992=APPLICATION_CONTEXT ( 'automotive_design' ) ;
#21996=CARTESIAN_POINT ( 'NONE',  ( 42.00000000000000711, 6.547216728259810428E-15, -1.617781153285278467E-30 ) ) ;
#22092=FACE_OUTER_BOUND ( 'NONE', #51832, .T. ) ;
#22144=ORIENTED_EDGE ( 'NONE', *, *, #13183, .T. ) ;
#22195=PRODUCT_DEFINITION ( 'UNKNOWN', '', #7877, #1597 ) ;
#22247=ORIENTED_EDGE ( 'NONE', *, *, #24762, .T. ) ;
#22291=ORIENTED_EDGE ( 'NONE', *, *, #59898, .F. ) ;
#22358=ORIENTED_EDGE ( 'NONE', *, *, #47810, .F. ) ;
#22435=VECTOR ( 'NONE', #29572, 1000.000000000000000 ) ;
#22609=DIRECTION ( 'NONE',  ( 1.000000000000000000, 1.558861125776144859E-16, -3.851859888774471706E-32 ) ) ;
#22621=LINE ( 'NONE', #21690, #41606 ) ;
#22639=EDGE_CURVE ( 'NONE', #32675, #58502, #21739, .T. ) ;
#22745=EDGE_CURVE ( 'NONE', #1357, #42003, #52384, .T. ) ;
#22784=FACE_OUTER_BOUND ( 'NONE', #21495, .T. ) ;
#22867=DIRECTION ( 'NONE',  ( 0.000000000000000000, 0.000000000000000000, 1.000000000000000000 ) ) ;
#22907=AXIS2_PLACEMENT_3D ( 'NONE', #28033, #47448, #9526 ) ;
#23044=EDGE_LOOP ( 'NONE', ( #19691, #9159 ) ) ;
#23084=CARTESIAN_POINT ( 'NONE',  ( 6.999999999999995559, 54.69470952477936976, 58.44237546506825964 ) ) ;
#23085=EDGE_CURVE ( 'NONE', #33072, #55726, #10974, .T. ) ;
#23136=ORIENTED_EDGE ( 'NONE', *, *, #40080, .F. ) ;
#23175=DIRECTION ( 'NONE',  ( -1.000000000000000000, -0.000000000000000000, -0.000000000000000000 ) ) ;
#23294=ORIENTED_EDGE ( 'NONE', *, *, #24397, .T. ) ;
#23316=DIRECTION ( 'NONE',  ( -1.000000000000000000, -3.673819061467147552E-16, 1.925929944387234758E-32 ) ) ;
#23333=CARTESIAN_POINT ( 'NONE',  ( 7.000000000000006217, -2.780326704359372228E-13, 80.00000000000001421 ) ) ;
#23461=EDGE_LOOP ( 'NONE', ( #30666, #38837, #58549, #3238 ) ) ;
#23465=DIRECTION ( 'NONE',  ( 2.168404344971009361E-16, -1.000000000000000000, 0.000000000000000000 ) ) ;
#23552=CARTESIAN_POINT ( 'NONE',  ( 42.00000000000000711, 16.00000000000000355, -1.502225356622044491E-30 ) ) ;
#23599=VECTOR ( 'NONE', #11823, 1000.000000000000000 ) ;
#23614=DIRECTION ( 'NONE',  ( 1.000000000000000000, 1.836909530733573776E-16, -1.925929944387235853E-32 ) ) ;
#23628=DIRECTION ( 'NONE',  ( 1.000000000000000000, 1.836909530733573776E-16, -1.925929944387235579E-32 ) ) ;
#23637=CARTESIAN_POINT ( 'NONE',  ( 45.00000000000001421, 0.000000000000000000, 0.000000000000000000 ) ) ;
#23645=EDGE_CURVE ( 'NONE', #38027, #3479, #27019, .T. ) ;
#23660=CYLINDRICAL_SURFACE ( 'NONE', #6135, 13.00000000000000178 ) ;
#23756=ORIENTED_EDGE ( 'NONE', *, *, #2821, .T. ) ;
#23763=CIRCLE ( 'NONE', #56789, 2.649999999999985700 ) ;
#23788=ADVANCED_FACE ( 'NONE', ( #18950 ), #4491, .F. ) ;
#23818=LINE ( 'NONE', #47940, #6490 ) ;
#24026=FACE_BOUND ( 'NONE', #1220, .T. ) ;
#24045=ADVANCED_FACE ( 'NONE', ( #46684 ), #41998, .T. ) ;
#24101=VERTEX_POINT ( 'NONE', #5271 ) ;
#24135=CIRCLE ( 'NONE', #40184, 13.00000000000000178 ) ;
#24286=VECTOR ( 'NONE', #3221, 1000.000000000000000 ) ;
#24342=ORIENTED_EDGE ( 'NONE', *, *, #7261, .T. ) ;
#24397=EDGE_CURVE ( 'NONE', #47270, #27605, #44045, .T. ) ;
#24404=( NAMED_UNIT ( * ) PLANE_ANGLE_UNIT ( ) SI_UNIT ( $, .RADIAN. ) );
#24418=DIRECTION ( 'NONE',  ( 0.000000000000000000, -0.7071067811865487940, 0.7071067811865461294 ) ) ;
#24460=ADVANCED_FACE ( 'NONE', ( #47845 ), #21794, .F. ) ;
#24466=CARTESIAN_POINT ( 'NONE',  ( 6.999999999999992895, 72.00000000000002842, -4.718528363748726964E-31 ) ) ;
#24485=CARTESIAN_POINT ( 'NONE',  ( 7.000000000000019540, -72.00000000000002842, 8.817456953860946444E-15 ) ) ;
#24601=ORIENTED_EDGE ( 'NONE', *, *, #47344, .F. ) ;
#24656=FACE_BOUND ( 'NONE', #8883, .T. ) ;
#24660=ADVANCED_FACE ( 'NONE', ( #45933 ), #41848, .F. ) ;
#24696=VERTEX_POINT ( 'NONE', #4503 ) ;
#24762=EDGE_CURVE ( 'NONE', #51041, #42003, #16064, .T. ) ;
#24835=( GEOMETRIC_REPRESENTATION_CONTEXT ( 3 ) GLOBAL_UNCERTAINTY_ASSIGNED_CONTEXT ( ( #9788 ) ) GLOBAL_UNIT_ASSIGNED_CONTEXT ( ( #33208, #24404, #47291 ) ) REPRESENTATION_CONTEXT ( 'NONE', 'WORKASPACE' ) );
#24999=EDGE_CURVE ( 'NONE', #59028, #49007, #36758, .T. ) ;
#25118=AXIS2_PLACEMENT_3D ( 'NONE', #979, #14793, #47684 ) ;
#25127=EDGE_LOOP ( 'NONE', ( #19369, #61844 ) ) ;
#25206=DIRECTION ( 'NONE',  ( -1.000000000000000000, -1.836909530733573776E-16, 1.925929944387235853E-32 ) ) ;
#25222=DIRECTION ( 'NONE',  ( 1.000000000000000000, 1.836909530733573776E-16, -1.925929944387235853E-32 ) ) ;
#25232=CARTESIAN_POINT ( 'NONE',  ( 10.00000000000001599, -58.44237546506844438, 54.69470952477916370 ) ) ;
#25240=CARTESIAN_POINT ( 'NONE',  ( 7.000000000000006217, -2.780326704359372228E-13, 80.00000000000001421 ) ) ;
#25259=AXIS2_PLACEMENT_3D ( 'NONE', #27331, #3501, #41768 ) ;
#25319=VERTEX_POINT ( 'NONE', #39392 ) ;
#25332=SHAPE_REPRESENTATION_RELATIONSHIP ( 'NONE' , 'NONE' ,  #6760, #4831 ) ;
#25644=CYLINDRICAL_SURFACE ( 'NONE', #34253, 2.649999999999992806 ) ;
#25675=DIRECTION ( 'NONE',  ( 0.000000000000000000, 0.7071067811865540120, -0.7071067811865409114 ) ) ;
#25722=DIRECTION ( 'NONE',  ( -1.000000000000000000, -1.836909530733573776E-16, -1.361838123766432833E-32 ) ) ;
#25804=CIRCLE ( 'NONE', #39843, 2.649999999999997691 ) ;
#25823=DIRECTION ( 'NONE',  ( -1.000000000000000000, -1.836909530733573776E-16, 1.925929944387234758E-32 ) ) ;
#25866=CARTESIAN_POINT ( 'NONE',  ( 6.999999999999995559, 56.56854249492450037, -56.56854249492312192 ) ) ;
#25895=CIRCLE ( 'NONE', #22907, 2.649999999999997691 ) ;
#25916=CARTESIAN_POINT ( 'NONE',  ( 42.00000000000000711, 19.00000000000000355, -1.617781153285278467E-30 ) ) ;
#25933=DIRECTION ( 'NONE',  ( -1.000000000000000000, -1.558861125776144859E-16, 3.851859888774471706E-32 ) ) ;
#25961=EDGE_CURVE ( 'NONE', #43795, #59028, #12057, .T. ) ;
#25962=FACE_OUTER_BOUND ( 'NONE', #13857, .T. ) ;
#26051=DIRECTION ( 'NONE',  ( 1.000000000000000000, 1.558861125776144859E-16, -3.851859888774471706E-32 ) ) ;
#26065=AXIS2_PLACEMENT_3D ( 'NONE', #58943, #14822, #58306 ) ;
#26090=EDGE_CURVE ( 'NONE', #51012, #58502, #34937, .T. ) ;
#26131=CARTESIAN_POINT ( 'NONE',  ( 7.000000000000006217, 1.285836671513502826E-15, -1.348150961071066192E-31 ) ) ;
#26140=DIRECTION ( 'NONE',  ( 0.000000000000000000, 0.000000000000000000, 1.000000000000000000 ) ) ;
#26172=CARTESIAN_POINT ( 'NONE',  ( 10.00000000000000533, -2.649999999999153033, -80.00000000000004263 ) ) ;
#26178=PRODUCT_CONTEXT ( 'NONE', #20346, 'mechanical' ) ;
#26352=DIRECTION ( 'NONE',  ( 0.000000000000000000, 1.000000000000000000, 0.000000000000000000 ) ) ;
#26426=FACE_OUTER_BOUND ( 'NONE', #18379, .T. ) ;
#26501=ORIENTED_EDGE ( 'NONE', *, *, #60867, .T. ) ;
#26514=FACE_OUTER_BOUND ( 'NONE', #7487, .T. ) ;
#26584=DIRECTION ( 'NONE',  ( 0.000000000000000000, 0.7071067811865395791, 0.7071067811865553443 ) ) ;
#26592=AXIS2_PLACEMENT_3D ( 'NONE', #26131, #25206, #40570 ) ;
#26731=FACE_BOUND ( 'NONE', #17754, .T. ) ;
#26972=CARTESIAN_POINT ( 'NONE',  ( 6.999999999999991118, 80.00000000000001421, 2.649999999999999467 ) ) ;
#27019=CIRCLE ( 'NONE', #16024, 2.649999999999999467 ) ;
#27044=DIRECTION ( 'NONE',  ( 1.836909530733573776E-16, -1.000000000000000000, 0.000000000000000000 ) ) ;
#27094=AXIS2_PLACEMENT_3D ( 'NONE', #33867, #30065, #34477 ) ;
#27120=DIRECTION ( 'NONE',  ( -1.000000000000000000, -1.836909530733573776E-16, 2.465190328815682145E-32 ) ) ;
#27135=DIRECTION ( 'NONE',  ( -1.000000000000000000, -1.836909530733573776E-16, 1.925929944387235853E-32 ) ) ;
#27201=EDGE_CURVE ( 'NONE', #39665, #57549, #25804, .T. ) ;
#27226=ADVANCED_FACE ( 'NONE', ( #22784 ), #33127, .T. ) ;
#27272=CARTESIAN_POINT ( 'NONE',  ( 6.999999999999995559, 58.44237546506807490, 54.69470952477956871 ) ) ;
#27331=CARTESIAN_POINT ( 'NONE',  ( 6.999999999999995559, 56.56854249492371878, 56.56854249492391062 ) ) ;
#27375=DIRECTION ( 'NONE',  ( -1.850371707708593823E-16, 1.000000000000000000, 0.000000000000000000 ) ) ;
#27381=DIRECTION ( 'NONE',  ( 0.000000000000000000, 0.7071067811865527908, -0.7071067811865421326 ) ) ;
#27383=DIRECTION ( 'NONE',  ( 0.000000000000000000, 1.000000000000000000, 0.000000000000000000 ) ) ;
#27391=DIRECTION ( 'NONE',  ( -1.000000000000000000, -5.380183451256491399E-17, -1.298891185607892835E-16 ) ) ;
#27445=DIRECTION ( 'NONE',  ( -1.000000000000000000, -0.000000000000000000, 1.925929944387235853E-32 ) ) ;
#27500=DIRECTION ( 'NONE',  ( 0.000000000000000000, -0.7071067811865461294, -0.7071067811865487940 ) ) ;
#27510=EDGE_CURVE ( 'NONE', #45271, #37250, #34901, .T. ) ;
#27522=ORIENTED_EDGE ( 'NONE', *, *, #20722, .F. ) ;
#27575=CIRCLE ( 'NONE', #16445, 85.00000000000001421 ) ;
#27605=VERTEX_POINT ( 'NONE', #38374 ) ;
#27679=CARTESIAN_POINT ( 'NONE',  ( 7.000000000000021316, -80.00000000000001421, -2.649999999999992806 ) ) ;
#27698=CARTESIAN_POINT ( 'NONE',  ( 7.000000000000016875, -56.56854249492331377, -56.56854249492430142 ) ) ;
#27868=VERTEX_POINT ( 'NONE', #23552 ) ;
#28033=CARTESIAN_POINT ( 'NONE',  ( 6.999999999999995559, 56.56854249492371878, 56.56854249492391062 ) ) ;
#28074=ORIENTED_EDGE ( 'NONE', *, *, #40545, .F. ) ;
#28100=ORIENTED_EDGE ( 'NONE', *, *, #49569, .T. ) ;
#28148=EDGE_LOOP ( 'NONE', ( #34235, #19632 ) ) ;
#28318=LINE ( 'NONE', #41518, #7658 ) ;
#28325=DIRECTION ( 'NONE',  ( -2.168404344971009361E-16, 1.000000000000000000, 0.000000000000000000 ) ) ;
#28463=ORIENTED_EDGE ( 'NONE', *, *, #13335, .F. ) ;
#28553=CIRCLE ( 'NONE', #61546, 18.99999999999999645 ) ;
#28653=AXIS2_PLACEMENT_3D ( 'NONE', #54311, #11754, #26140 ) ;
#28657=AXIS2_PLACEMENT_3D ( 'NONE', #2571, #49891, #6625 ) ;
#28669=CARTESIAN_POINT ( 'NONE',  ( 42.00000000000000711, -15.99999999999998934, 1.959434878635763159E-15 ) ) ;
#28811=CARTESIAN_POINT ( 'NONE',  ( 6.999999999999995559, 56.56854249492371878, 56.56854249492391062 ) ) ;
#28825=CIRCLE ( 'NONE', #8842, 85.00000000000001421 ) ;
#28930=VECTOR ( 'NONE', #3842, 1000.000000000000000 ) ;
#28931=ORIENTED_EDGE ( 'NONE', *, *, #61718, .F. ) ;
#29143=CARTESIAN_POINT ( 'NONE',  ( 10.00000000000001599, -58.44237546506767700, -54.69470952477997372 ) ) ;
#29346=CARTESIAN_POINT ( 'NONE',  ( 7.000000000000016875, -58.44237546506844438, 54.69470952477915660 ) ) ;
#29380=EDGE_CURVE ( 'NONE', #33929, #12652, #49907, .T. ) ;
#29416=ADVANCED_FACE ( 'NONE', ( #61821 ), #43384, .F. ) ;
#29444=EDGE_CURVE ( 'NONE', #24101, #3387, #25895, .T. ) ;
#29522=ORIENTED_EDGE ( 'NONE', *, *, #55338, .F. ) ;
#29535=AXIS2_PLACEMENT_3D ( 'NONE', #35717, #40731, #1004 ) ;
#29572=DIRECTION ( 'NONE',  ( -1.000000000000000000, -1.836909530733580185E-16, 1.836909530733574022E-16 ) ) ;
#29653=DIRECTION ( 'NONE',  ( -1.000000000000000000, -1.836909530733573776E-16, 1.925929944387235853E-32 ) ) ;
#29659=ORIENTED_EDGE ( 'NONE', *, *, #24762, .F. ) ;
#29661=DIRECTION ( 'NONE',  ( 0.000000000000000000, 0.000000000000000000, -1.000000000000000000 ) ) ;
#29688=EDGE_LOOP ( 'NONE', ( #7452, #44705, #20223, #47006 ) ) ;
#29735=DIRECTION ( 'NONE',  ( 0.000000000000000000, 0.000000000000000000, 1.000000000000000000 ) ) ;
#29766=VECTOR ( 'NONE', #11937, 1000.000000000000000 ) ;
#29856=CYLINDRICAL_SURFACE ( 'NONE', #31697, 75.00000000000001421 ) ;
#29945=DIRECTION ( 'NONE',  ( -1.000000000000000000, -5.380183451256491399E-17, -1.298891185607892835E-16 ) ) ;
#29977=EDGE_LOOP ( 'NONE', ( #59428, #22291, #36786, #30935 ) ) ;
#30065=DIRECTION ( 'NONE',  ( 1.000000000000000000, 1.558861125776144859E-16, -3.851859888774471706E-32 ) ) ;
#30116=EDGE_LOOP ( 'NONE', ( #39510, #6600, #32923, #36812 ) ) ;
#30155=EDGE_LOOP ( 'NONE', ( #56149, #17509, #1845, #44075 ) ) ;
#30187=ORIENTED_EDGE ( 'NONE', *, *, #36032, .F. ) ;
#30219=ORIENTED_EDGE ( 'NONE', *, *, #59584, .T. ) ;
#30226=ORIENTED_EDGE ( 'NONE', *, *, #1450, .F. ) ;
#30267=ADVANCED_FACE ( 'NONE', ( #25962 ), #25644, .F. ) ;
#30358=DIRECTION ( 'NONE',  ( -1.000000000000000000, -3.135800716341471541E-16, -1.298891185607920445E-16 ) ) ;
#30471=AXIS2_PLACEMENT_3D ( 'NONE', #10557, #29653, #5821 ) ;
#30519=VECTOR ( 'NONE', #27445, 1000.000000000000000 ) ;
#30532=( LENGTH_UNIT ( ) NAMED_UNIT ( * ) SI_UNIT ( .MILLI., .METRE. ) );
#30578=ORIENTED_EDGE ( 'NONE', *, *, #54648, .F. ) ;
#30580=CARTESIAN_POINT ( 'NONE',  ( 9.999999999999989342, 85.00000000000001421, 1.040949779275250495E-14 ) ) ;
#30618=ORIENTED_EDGE ( 'NONE', *, *, #48931, .F. ) ;
#30661=DIRECTION ( 'NONE',  ( 1.850371707708593823E-16, -1.000000000000000000, 0.000000000000000000 ) ) ;
#30666=ORIENTED_EDGE ( 'NONE', *, *, #53614, .F. ) ;
#30676=ORIENTED_EDGE ( 'NONE', *, *, #16729, .T. ) ;
#30684=ORIENTED_EDGE ( 'NONE', *, *, #37010, .F. ) ;
#30815=DIRECTION ( 'NONE',  ( 1.000000000000000000, 1.836909530733573776E-16, -1.925929944387235579E-32 ) ) ;
#30870=DIRECTION ( 'NONE',  ( 0.000000000000000000, -0.7071067811865487940, 0.7071067811865461294 ) ) ;
#30914=ORIENTED_EDGE ( 'NONE', *, *, #47344, .T. ) ;
#30916=EDGE_CURVE ( 'NONE', #35841, #24101, #51063, .T. ) ;
#30935=ORIENTED_EDGE ( 'NONE', *, *, #54648, .T. ) ;
#31000=ORIENTED_EDGE ( 'NONE', *, *, #12325, .F. ) ;
#31172=CYLINDRICAL_SURFACE ( 'NONE', #16957, 2.649999999999992806 ) ;
#31258=ORIENTED_EDGE ( 'NONE', *, *, #35694, .T. ) ;
#31441=ORIENTED_EDGE ( 'NONE', *, *, #6161, .T. ) ;
#31450=CIRCLE ( 'NONE', #4456, 2.649999999999985700 ) ;
#31452=ORIENTED_EDGE ( 'NONE', *, *, #55338, .T. ) ;
#31465=ADVANCED_FACE ( 'NONE', ( #20582 ), #33461, .F. ) ;
#31545=ORIENTED_EDGE ( 'NONE', *, *, #53614, .T. ) ;
#31572=DIRECTION ( 'NONE',  ( -1.000000000000000000, -3.135800716341489291E-16, 1.298891185607901956E-16 ) ) ;
#31692=VERTEX_POINT ( 'NONE', #30580 ) ;
#31697=AXIS2_PLACEMENT_3D ( 'NONE', #20464, #39595, #48656 ) ;
#31748=CARTESIAN_POINT ( 'NONE',  ( 6.999999999999995559, 54.69470952477936976, 58.44237546506825964 ) ) ;
#31912=CARTESIAN_POINT ( 'NONE',  ( 42.00000000000000711, -18.99999999999998934, 2.326828918379968998E-15 ) ) ;
#31913=DIRECTION ( 'NONE',  ( 1.000000000000000000, 1.836909530733573776E-16, -1.925929944387235579E-32 ) ) ;
#31914=EDGE_LOOP ( 'NONE', ( #18659, #15117 ) ) ;
#31969=AXIS2_PLACEMENT_3D ( 'NONE', #49159, #53835, #30661 ) ;
#31983=DIRECTION ( 'NONE',  ( -1.000000000000000000, -5.380183451256670742E-17, 1.298891185607911324E-16 ) ) ;
#32076=DIRECTION ( 'NONE',  ( -1.826024711554534160E-16, 1.000000000000000000, 0.000000000000000000 ) ) ;
#32097=FACE_OUTER_BOUND ( 'NONE', #1693, .T. ) ;
#32115=DIRECTION ( 'NONE',  ( 0.000000000000000000, 0.000000000000000000, -1.000000000000000000 ) ) ;
#32131=CYLINDRICAL_SURFACE ( 'NONE', #40514, 2.649999999999992806 ) ;
#32203=DIRECTION ( 'NONE',  ( 1.836909530733573776E-16, -1.000000000000000000, 0.000000000000000000 ) ) ;
#32225=FACE_OUTER_BOUND ( 'NONE', #40881, .T. ) ;
#32227=FACE_OUTER_BOUND ( 'NONE', #38327, .T. ) ;
#32334=CARTESIAN_POINT ( 'NONE',  ( 45.00000000000001421, 7.805869035311033600E-47, 13.00000000000000178 ) ) ;
#32351=DIRECTION ( 'NONE',  ( -1.000000000000000000, -1.836909530733573776E-16, 1.361838123766442686E-32 ) ) ;
#32425=CARTESIAN_POINT ( 'NONE',  ( 7.000000000000021316, -80.00000000000001421, -1.954818893553044610E-31 ) ) ;
#32428=ORIENTED_EDGE ( 'NONE', *, *, #10966, .F. ) ;
#32432=DIRECTION ( 'NONE',  ( -1.000000000000000000, -3.135800716341471541E-16, -1.298891185607920445E-16 ) ) ;
#32636=EDGE_CURVE ( 'NONE', #49531, #31692, #45399, .T. ) ;
#32647=DIRECTION ( 'NONE',  ( 0.000000000000000000, -1.047444401652941269E-14, 1.000000000000000000 ) ) ;
#32675=VERTEX_POINT ( 'NONE', #45689 ) ;
#32698=DIRECTION ( 'NONE',  ( -1.000000000000000000, -1.836909530733573776E-16, 1.925929944387235853E-32 ) ) ;
#32883=ORIENTED_EDGE ( 'NONE', *, *, #22639, .F. ) ;
#32923=ORIENTED_EDGE ( 'NONE', *, *, #8397, .F. ) ;
#33012=VERTEX_POINT ( 'NONE', #26172 ) ;
#33072=VERTEX_POINT ( 'NONE', #6112 ) ;
#33127=CYLINDRICAL_SURFACE ( 'NONE', #43865, 85.00000000000001421 ) ;
#33193=DIRECTION ( 'NONE',  ( 0.000000000000000000, 0.000000000000000000, 1.000000000000000000 ) ) ;
#33208=( LENGTH_UNIT ( ) NAMED_UNIT ( * ) SI_UNIT ( .MILLI., .METRE. ) );
#33233=AXIS2_PLACEMENT_3D ( 'NONE', #17630, #32351, #41455 ) ;
#33461=CYLINDRICAL_SURFACE ( 'NONE', #41335, 2.649999999999992806 ) ;
#33466=VECTOR ( 'NONE', #46590, 1000.000000000000000 ) ;
#33750=DIRECTION ( 'NONE',  ( 0.000000000000000000, 3.491481338843138088E-15, -1.000000000000000000 ) ) ;
#33799=CARTESIAN_POINT ( 'NONE',  ( 45.00000000000001421, 0.000000000000000000, 0.000000000000000000 ) ) ;
#33857=ORIENTED_EDGE ( 'NONE', *, *, #30916, .F. ) ;
#33867=CARTESIAN_POINT ( 'NONE',  ( 42.00000000000000711, 0.000000000000000000, 0.000000000000000000 ) ) ;
#33929=VERTEX_POINT ( 'NONE', #20270 ) ;
#33977=ORIENTED_EDGE ( 'NONE', *, *, #56001, .T. ) ;
#33982=CARTESIAN_POINT ( 'NONE',  ( 7.000000000000016875, -56.56854249492331377, -56.56854249492430142 ) ) ;
#34008=DIRECTION ( 'NONE',  ( 1.000000000000000000, 1.836909530733573776E-16, -1.925929944387235853E-32 ) ) ;
#34057=DIRECTION ( 'NONE',  ( 1.836766033387207149E-16, -1.000000000000000000, 0.000000000000000000 ) ) ;
#34094=CYLINDRICAL_SURFACE ( 'NONE', #38029, 2.649999999999992806 ) ;
#34107=PLANE ( 'NONE',  #55155 ) ;
#34235=ORIENTED_EDGE ( 'NONE', *, *, #25961, .T. ) ;
#34253=AXIS2_PLACEMENT_3D ( 'NONE', #46025, #39785, #20955 ) ;
#34296=EDGE_CURVE ( 'NONE', #47270, #3479, #10169, .T. ) ;
#34318=EDGE_CURVE ( 'NONE', #31692, #1874, #14269, .T. ) ;
#34398=CYLINDRICAL_SURFACE ( 'NONE', #54480, 2.649999999999992806 ) ;
#34430=ORIENTED_EDGE ( 'NONE', *, *, #4309, .T. ) ;
#34477=DIRECTION ( 'NONE',  ( -1.558861125776144859E-16, 1.000000000000000000, 0.000000000000000000 ) ) ;
#34480=CIRCLE ( 'NONE', #35471, 15.99999999999999645 ) ;
#34653=CARTESIAN_POINT ( 'NONE',  ( 6.999999999999995559, 58.44237546506882808, -54.69470952477875869 ) ) ;
#34702=CIRCLE ( 'NONE', #37713, 13.00000000000000178 ) ;
#34776=AXIS2_PLACEMENT_3D ( 'NONE', #52219, #47545, #14968 ) ;
#34786=FACE_BOUND ( 'NONE', #13092, .T. ) ;
#34793=AXIS2_PLACEMENT_3D ( 'NONE', #3042, #41294, #17465 ) ;
#34901=CIRCLE ( 'NONE', #56863, 2.649999999999992806 ) ;
#34918=ORIENTED_EDGE ( 'NONE', *, *, #40545, .T. ) ;
#34937=CIRCLE ( 'NONE', #20933, 18.99999999999999645 ) ;
#34972=DIRECTION ( 'NONE',  ( 3.273063162220391312E-16, -1.000000000000000000, -5.236901059552626099E-15 ) ) ;
#34999=FACE_BOUND ( 'NONE', #31914, .T. ) ;
#35291=CIRCLE ( 'NONE', #57242, 75.00000000000001421 ) ;
#35324=ADVANCED_FACE ( 'NONE', ( #14997, #19380 ), #34107, .T. ) ;
#35361=DIRECTION ( 'NONE',  ( -1.000000000000000000, -1.836909530733573776E-16, 1.925929944387235853E-32 ) ) ;
#35429=DIRECTION ( 'NONE',  ( 0.000000000000000000, 0.000000000000000000, 1.000000000000000000 ) ) ;
#35468=ORIENTED_EDGE ( 'NONE', *, *, #7334, .T. ) ;
#35471=AXIS2_PLACEMENT_3D ( 'NONE', #21996, #13215, #2557 ) ;
#35539=CARTESIAN_POINT ( 'NONE',  ( 45.00000000000001421, 0.000000000000000000, 0.000000000000000000 ) ) ;
#35562=AXIS2_PLACEMENT_3D ( 'NONE', #40565, #30815, #32076 ) ;
#35694=EDGE_CURVE ( 'NONE', #18038, #45374, #5171, .T. ) ;
#35717=CARTESIAN_POINT ( 'NONE',  ( 10.00000000000001599, -56.56854249492410958, 56.56854249492351983 ) ) ;
#35841=VERTEX_POINT ( 'NONE', #36118 ) ;
#35844=FACE_BOUND ( 'NONE', #35950, .T. ) ;
#35878=ORIENTED_EDGE ( 'NONE', *, *, #59116, .T. ) ;
#35923=ORIENTED_EDGE ( 'NONE', *, *, #2917, .T. ) ;
#35950=EDGE_LOOP ( 'NONE', ( #43521, #32428 ) ) ;
#36016=EDGE_LOOP ( 'NONE', ( #31000, #31452, #40625, #8888 ) ) ;
#36032=EDGE_CURVE ( 'NONE', #59028, #43795, #2753, .T. ) ;
#36041=EDGE_LOOP ( 'NONE', ( #30676, #46432 ) ) ;
#36068=CARTESIAN_POINT ( 'NONE',  ( 7.000000000000021316, -80.00000000000001421, -2.649999999999999467 ) ) ;
#36103=ORIENTED_EDGE ( 'NONE', *, *, #59584, .F. ) ;
#36118=CARTESIAN_POINT ( 'NONE',  ( 9.999999999999994671, 58.44237546506807490, 54.69470952477956871 ) ) ;
#36242=EDGE_CURVE ( 'NONE', #49531, #3017, #55724, .T. ) ;
#36243=DIRECTION ( 'NONE',  ( 0.000000000000000000, 0.000000000000000000, 1.000000000000000000 ) ) ;
#36245=DIRECTION ( 'NONE',  ( -1.807003620809173399E-16, 1.000000000000000000, 0.000000000000000000 ) ) ;
#36265=DIRECTION ( 'NONE',  ( 0.000000000000000000, 0.000000000000000000, -1.000000000000000000 ) ) ;
#36295=FACE_OUTER_BOUND ( 'NONE', #19401, .T. ) ;
#36305=CARTESIAN_POINT ( 'NONE',  ( 10.00000000000002132, -85.00000000000001421, -1.925929944387237167E-31 ) ) ;
#36396=ORIENTED_EDGE ( 'NONE', *, *, #55140, .F. ) ;
#36547=CIRCLE ( 'NONE', #15571, 2.649999999999992806 ) ;
#36551=CIRCLE ( 'NONE', #38569, 2.649999999999999467 ) ;
#36741=ORIENTED_EDGE ( 'NONE', *, *, #26090, .F. ) ;
#36758=LINE ( 'NONE', #46461, #59054 ) ;
#36785=ORIENTED_EDGE ( 'NONE', *, *, #48647, .F. ) ;
#36786=ORIENTED_EDGE ( 'NONE', *, *, #851, .T. ) ;
#36812=ORIENTED_EDGE ( 'NONE', *, *, #55343, .F. ) ;
#36878=ADVANCED_FACE ( 'NONE', ( #7976 ), #46216, .T. ) ;
#36890=DIRECTION ( 'NONE',  ( 0.000000000000000000, 0.7071067811865382469, 0.7071067811865566766 ) ) ;
#36940=DIRECTION ( 'NONE',  ( -1.807003620809173399E-16, 1.000000000000000000, 0.000000000000000000 ) ) ;
#37010=EDGE_CURVE ( 'NONE', #45271, #50728, #28318, .T. ) ;
#37054=CARTESIAN_POINT ( 'NONE',  ( 30.00000000000000711, 16.00000000000000000, -1.386669559958810165E-30 ) ) ;
#37080=ADVANCED_FACE ( 'NONE', ( #38364 ), #29856, .T. ) ;
#37146=CARTESIAN_POINT ( 'NONE',  ( 7.000000000000016875, -56.56854249492331377, -56.56854249492430142 ) ) ;
#37169=FACE_OUTER_BOUND ( 'NONE', #10659, .T. ) ;
#37219=DIRECTION ( 'NONE',  ( -1.558861125776144859E-16, 1.000000000000000000, 0.000000000000000000 ) ) ;
#37250=VERTEX_POINT ( 'NONE', #18244 ) ;
#37267=ORIENTED_EDGE ( 'NONE', *, *, #1450, .T. ) ;
#37514=ORIENTED_EDGE ( 'NONE', *, *, #38598, .F. ) ;
#37552=FACE_OUTER_BOUND ( 'NONE', #17573, .T. ) ;
#37554=VERTEX_POINT ( 'NONE', #48139 ) ;
#37713=AXIS2_PLACEMENT_3D ( 'NONE', #7225, #26051, #26352 ) ;
#37748=CARTESIAN_POINT ( 'NONE',  ( 7.000000000000019540, -72.00000000000002842, 8.817456953860944867E-15 ) ) ;
#37770=DIRECTION ( 'NONE',  ( 3.273063162220399693E-16, -1.000000000000000000, -5.236901059552639509E-15 ) ) ;
#37781=AXIS2_PLACEMENT_3D ( 'NONE', #53225, #48534, #29735 ) ;
#37812=AXIS2_PLACEMENT_3D ( 'NONE', #20998, #39830, #57949 ) ;
#38017=CARTESIAN_POINT ( 'NONE',  ( 45.00000000000001421, 2.163354392537210416E-30, 75.00000000000001421 ) ) ;
#38027=VERTEX_POINT ( 'NONE', #16287 ) ;
#38029=AXIS2_PLACEMENT_3D ( 'NONE', #53465, #57225, #43184 ) ;
#38063=ORIENTED_EDGE ( 'NONE', *, *, #52505, .T. ) ;
#38327=EDGE_LOOP ( 'NONE', ( #30684, #26, #54858, #21927 ) ) ;
#38328=CYLINDRICAL_SURFACE ( 'NONE', #2659, 72.00000000000002842 ) ;
#38364=FACE_OUTER_BOUND ( 'NONE', #15112, .T. ) ;
#38374=CARTESIAN_POINT ( 'NONE',  ( 10.00000000000000533, -2.650000000000270362, 80.00000000000000000 ) ) ;
#38431=VERTEX_POINT ( 'NONE', #61095 ) ;
#38569=AXIS2_PLACEMENT_3D ( 'NONE', #13378, #41897, #36265 ) ;
#38598=EDGE_CURVE ( 'NONE', #11927, #10882, #42759, .T. ) ;
#38604=AXIS2_PLACEMENT_3D ( 'NONE', #3304, #27135, #36243 ) ;
#38620=VERTEX_POINT ( 'NONE', #55400 ) ;
#38792=ORIENTED_EDGE ( 'NONE', *, *, #25961, .F. ) ;
#38798=FACE_OUTER_BOUND ( 'NONE', #43802, .T. ) ;
#38837=ORIENTED_EDGE ( 'NONE', *, *, #48647, .T. ) ;
#38985=CARTESIAN_POINT ( 'NONE',  ( 30.00000000000001066, 4.342925291379521108E-15, -1.386669559958810165E-30 ) ) ;
#39086=EDGE_LOOP ( 'NONE', ( #43197, #4063 ) ) ;
#39089=FACE_BOUND ( 'NONE', #4236, .T. ) ;
#39171=ORIENTED_EDGE ( 'NONE', *, *, #21933, .T. ) ;
#39392=CARTESIAN_POINT ( 'NONE',  ( 45.00000000000001421, 1.592040838891559293E-15, -13.00000000000000178 ) ) ;
#39502=AXIS2_PLACEMENT_3D ( 'NONE', #51396, #22609, #45507 ) ;
#39510=ORIENTED_EDGE ( 'NONE', *, *, #23085, .T. ) ;
#39595=DIRECTION ( 'NONE',  ( -1.000000000000000000, -0.000000000000000000, -0.000000000000000000 ) ) ;
#39635=CIRCLE ( 'NONE', #26592, 85.00000000000001421 ) ;
#39665=VERTEX_POINT ( 'NONE', #9659 ) ;
#39685=CIRCLE ( 'NONE', #28657, 2.649999999999999467 ) ;
#39767=DIRECTION ( 'NONE',  ( 1.836766033387207149E-16, -1.000000000000000000, 0.000000000000000000 ) ) ;
#39776=AXIS2_PLACEMENT_3D ( 'NONE', #20982, #54783, #11918 ) ;
#39785=DIRECTION ( 'NONE',  ( -1.000000000000000000, -3.673819061467147552E-16, 1.925929944387234758E-32 ) ) ;
#39813=CARTESIAN_POINT ( 'NONE',  ( 7.000000000000016875, -56.56854249492331377, -56.56854249492430142 ) ) ;
#39830=DIRECTION ( 'NONE',  ( -1.000000000000000000, -1.836909530733573776E-16, 1.925929944387235853E-32 ) ) ;
#39843=AXIS2_PLACEMENT_3D ( 'NONE', #60666, #13094, #17784 ) ;
#40006=DIRECTION ( 'NONE',  ( -1.000000000000000000, -5.380183451256670742E-17, 1.298891185607911324E-16 ) ) ;
#40080=EDGE_CURVE ( 'NONE', #55180, #50728, #43717, .T. ) ;
#40149=CIRCLE ( 'NONE', #57071, 2.649999999999999467 ) ;
#40184=AXIS2_PLACEMENT_3D ( 'NONE', #58434, #54048, #49366 ) ;
#40316=EDGE_CURVE ( 'NONE', #38620, #1988, #7972, .T. ) ;
#40334=ORIENTED_EDGE ( 'NONE', *, *, #55372, .T. ) ;
#40352=EDGE_LOOP ( 'NONE', ( #28931, #47241, #44056, #40666 ) ) ;
#40514=AXIS2_PLACEMENT_3D ( 'NONE', #18348, #8603, #4817 ) ;
#40517=CARTESIAN_POINT ( 'NONE',  ( 30.00000000000001066, 4.342925291379521108E-15, -1.386669559958810165E-30 ) ) ;
#40545=EDGE_CURVE ( 'NONE', #10882, #11927, #39685, .T. ) ;
#40565=CARTESIAN_POINT ( 'NONE',  ( 30.00000000000001066, 4.342925291379521108E-15, -1.386669559958810165E-30 ) ) ;
#40570=DIRECTION ( 'NONE',  ( 1.836766033387207149E-16, -1.000000000000000000, 0.000000000000000000 ) ) ;
#40625=ORIENTED_EDGE ( 'NONE', *, *, #55343, .T. ) ;
#40666=ORIENTED_EDGE ( 'NONE', *, *, #44992, .F. ) ;
#40731=DIRECTION ( 'NONE',  ( -1.000000000000000000, -1.836909530733573776E-16, 1.103352205049209901E-32 ) ) ;
#40790=CIRCLE ( 'NONE', #9868, 2.649999999999999467 ) ;
#40881=EDGE_LOOP ( 'NONE', ( #53870, #54080, #21827, #57564 ) ) ;
#40936=CIRCLE ( 'NONE', #21906, 2.649999999999997691 ) ;
#40969=CARTESIAN_POINT ( 'NONE',  ( 7.000000000000016875, -58.44237546506844438, 54.69470952477916370 ) ) ;
#41016=CARTESIAN_POINT ( 'NONE',  ( 7.000000000000005329, 2.650000000000838796, -79.99999999999998579 ) ) ;
#41040=LINE ( 'NONE', #56320, #9827 ) ;
#41125=ORIENTED_EDGE ( 'NONE', *, *, #35694, .F. ) ;
#41170=ORIENTED_EDGE ( 'NONE', *, *, #851, .F. ) ;
#41199=VECTOR ( 'NONE', #25222, 1000.000000000000000 ) ;
#41234=ADVANCED_FACE ( 'NONE', ( #47711 ), #38328, .F. ) ;
#41294=DIRECTION ( 'NONE',  ( -1.000000000000000000, -1.558861125776144859E-16, 3.851859888774471706E-32 ) ) ;
#41335=AXIS2_PLACEMENT_3D ( 'NONE', #9630, #57846, #29661 ) ;
#41444=LINE ( 'NONE', #37054, #52575 ) ;
#41455=DIRECTION ( 'NONE',  ( 0.000000000000000000, -0.7071067811865461294, -0.7071067811865487940 ) ) ;
#41505=CARTESIAN_POINT ( 'NONE',  ( 6.999999999999991118, 80.00000000000001421, -7.414830285890871171E-32 ) ) ;
#41518=CARTESIAN_POINT ( 'NONE',  ( 6.999999999999995559, 54.69470952478017978, -58.44237546506749226 ) ) ;
#41606=VECTOR ( 'NONE', #12013, 1000.000000000000000 ) ;
#41610=PLANE ( 'NONE',  #12633 ) ;
#41638=ORIENTED_EDGE ( 'NONE', *, *, #48931, .T. ) ;
#41674=CARTESIAN_POINT ( 'NONE',  ( 30.00000000000001421, -15.99999999999999289, 1.959434878635763159E-15 ) ) ;
#41768=DIRECTION ( 'NONE',  ( 0.000000000000000000, -0.7071067811865487940, 0.7071067811865461294 ) ) ;
#41790=ORIENTED_EDGE ( 'NONE', *, *, #40316, .T. ) ;
#41848=CYLINDRICAL_SURFACE ( 'NONE', #14026, 2.649999999999992806 ) ;
#41873=VECTOR ( 'NONE', #31572, 1000.000000000000000 ) ;
#41897=DIRECTION ( 'NONE',  ( -1.000000000000000000, -3.673819061467147552E-16, 1.925929944387234758E-32 ) ) ;
#41998=CYLINDRICAL_SURFACE ( 'NONE', #51993, 75.00000000000001421 ) ;
#42003=VERTEX_POINT ( 'NONE', #60403 ) ;
#42121=LINE ( 'NONE', #27679, #17092 ) ;
#42187=DIRECTION ( 'NONE',  ( -1.000000000000000000, -1.836909530733580185E-16, 1.836909530733574022E-16 ) ) ;
#42379=FACE_OUTER_BOUND ( 'NONE', #60331, .T. ) ;
#42547=CARTESIAN_POINT ( 'NONE',  ( 7.000000000000007105, -2.649999999999161027, -80.00000000000004263 ) ) ;
#42759=CIRCLE ( 'NONE', #39776, 2.649999999999999467 ) ;
#42776=CARTESIAN_POINT ( 'NONE',  ( 9.999999999999989342, 85.00000000000001421, 1.040949779275250495E-14 ) ) ;
#42814=ORIENTED_EDGE ( 'NONE', *, *, #2917, .F. ) ;
#42880=EDGE_LOOP ( 'NONE', ( #30187, #1544, #48235, #9981 ) ) ;
#43043=AXIS2_PLACEMENT_3D ( 'NONE', #38985, #23628, #28325 ) ;
#43126=AXIS2_PLACEMENT_3D ( 'NONE', #15682, #53247, #43577 ) ;
#43184=DIRECTION ( 'NONE',  ( -3.273063162220399693E-16, 1.000000000000000000, 1.047380211910527902E-14 ) ) ;
#43197=ORIENTED_EDGE ( 'NONE', *, *, #43200, .T. ) ;
#43200=EDGE_CURVE ( 'NONE', #24696, #20064, #14904, .T. ) ;
#43245=VERTEX_POINT ( 'NONE', #25232 ) ;
#43384=CYLINDRICAL_SURFACE ( 'NONE', #6863, 2.649999999999992806 ) ;
#43487=CARTESIAN_POINT ( 'NONE',  ( 45.00000000000001421, 0.000000000000000000, 75.00000000000001421 ) ) ;
#43489=AXIS2_PLACEMENT_3D ( 'NONE', #17828, #2778, #8401 ) ;
#43509=DIRECTION ( 'NONE',  ( 1.000000000000000000, 1.558861125776144859E-16, -3.851859888774471706E-32 ) ) ;
#43521=ORIENTED_EDGE ( 'NONE', *, *, #23645, .F. ) ;
#43528=DIRECTION ( 'NONE',  ( 0.000000000000000000, 0.000000000000000000, 1.000000000000000000 ) ) ;
#43577=DIRECTION ( 'NONE',  ( 0.000000000000000000, 0.000000000000000000, 1.000000000000000000 ) ) ;
#43675=ORIENTED_EDGE ( 'NONE', *, *, #1045, .F. ) ;
#43717=CIRCLE ( 'NONE', #21642, 2.649999999999997691 ) ;
#43795=VERTEX_POINT ( 'NONE', #7264 ) ;
#43802=EDGE_LOOP ( 'NONE', ( #48191, #30219, #20762, #45226 ) ) ;
#43865=AXIS2_PLACEMENT_3D ( 'NONE', #19328, #56897, #34057 ) ;
#44045=CIRCLE ( 'NONE', #12995, 2.649999999999985700 ) ;
#44051=DIRECTION ( 'NONE',  ( 0.000000000000000000, 1.000000000000000000, 0.000000000000000000 ) ) ;
#44056=ORIENTED_EDGE ( 'NONE', *, *, #50491, .T. ) ;
#44075=ORIENTED_EDGE ( 'NONE', *, *, #52051, .F. ) ;
#44076=DIRECTION ( 'NONE',  ( -1.000000000000000000, -1.836909530733573776E-16, 1.925929944387235853E-32 ) ) ;
#44273=ORIENTED_EDGE ( 'NONE', *, *, #4020, .T. ) ;
#44352=VERTEX_POINT ( 'NONE', #7077 ) ;
#44369=DIRECTION ( 'NONE',  ( 0.000000000000000000, 0.7071067811865421326, 0.7071067811865527908 ) ) ;
#44688=CIRCLE ( 'NONE', #28653, 72.00000000000002842 ) ;
#44705=ORIENTED_EDGE ( 'NONE', *, *, #8320, .T. ) ;
#44707=FACE_BOUND ( 'NONE', #28148, .T. ) ;
#44751=ORIENTED_EDGE ( 'NONE', *, *, #52051, .T. ) ;
#44874=ORIENTED_EDGE ( 'NONE', *, *, #59864, .T. ) ;
#44942=FACE_BOUND ( 'NONE', #50177, .T. ) ;
#44992=EDGE_CURVE ( 'NONE', #47400, #51041, #7151, .T. ) ;
#45038=LINE ( 'NONE', #16825, #23599 ) ;
#45070=DIRECTION ( 'NONE',  ( 0.000000000000000000, 1.000000000000000000, 0.000000000000000000 ) ) ;
#45225=ADVANCED_FACE ( 'NONE', ( #38798 ), #34094, .F. ) ;
#45226=ORIENTED_EDGE ( 'NONE', *, *, #55372, .F. ) ;
#45253=FACE_BOUND ( 'NONE', #739, .T. ) ;
#45271=VERTEX_POINT ( 'NONE', #48180 ) ;
#45292=ORIENTED_EDGE ( 'NONE', *, *, #24397, .F. ) ;
#45374=VERTEX_POINT ( 'NONE', #59713 ) ;
#45399=CIRCLE ( 'NONE', #13370, 85.00000000000001421 ) ;
#45413=ADVANCED_FACE ( 'NONE', ( #26514 ), #58772, .F. ) ;
#45507=DIRECTION ( 'NONE',  ( 0.000000000000000000, 1.000000000000000000, 0.000000000000000000 ) ) ;
#45518=DIRECTION ( 'NONE',  ( 2.168404344971009361E-16, -1.000000000000000000, 0.000000000000000000 ) ) ;
#45689=CARTESIAN_POINT ( 'NONE',  ( 30.00000000000001421, -18.99999999999999289, 2.326828918379969393E-15 ) ) ;
#45752=CARTESIAN_POINT ( 'NONE',  ( 6.999999999999991118, 80.00000000000001421, -7.414830285890871171E-32 ) ) ;
#45788=VECTOR ( 'NONE', #48690, 1000.000000000000000 ) ;
#45814=PRODUCT_DEFINITION_SHAPE ( 'NONE', 'NONE',  #22195 ) ;
#45827=CIRCLE ( 'NONE', #11792, 72.00000000000002842 ) ;
#45933=FACE_OUTER_BOUND ( 'NONE', #40352, .T. ) ;
#45969=DIRECTION ( 'NONE',  ( -1.000000000000000000, -3.135800716341489291E-16, 1.298891185607901956E-16 ) ) ;
#46025=CARTESIAN_POINT ( 'NONE',  ( 7.000000000000021316, -80.00000000000001421, -1.954818893553044610E-31 ) ) ;
#46164=DIRECTION ( 'NONE',  ( -1.000000000000000000, -1.836909530733573776E-16, 2.465190328815655050E-32 ) ) ;
#46216=CYLINDRICAL_SURFACE ( 'NONE', #50679, 85.00000000000001421 ) ;
#46270=LINE ( 'NONE', #13365, #30519 ) ;
#46280=EDGE_CURVE ( 'NONE', #50174, #51012, #60961, .T. ) ;
#46374=ORIENTED_EDGE ( 'NONE', *, *, #34318, .T. ) ;
#46378=CARTESIAN_POINT ( 'NONE',  ( 45.00000000000001421, 0.000000000000000000, 0.000000000000000000 ) ) ;
#46432=ORIENTED_EDGE ( 'NONE', *, *, #29380, .T. ) ;
#46461=CARTESIAN_POINT ( 'NONE',  ( 6.999999999999991118, 80.00000000000001421, -2.649999999999992806 ) ) ;
#46485=DIRECTION ( 'NONE',  ( 1.000000000000000000, 1.836909530733573776E-16, -1.925929944387235579E-32 ) ) ;
#46556=ORIENTED_EDGE ( 'NONE', *, *, #2157, .T. ) ;
#46557=CIRCLE ( 'NONE', #29535, 2.649999999999992806 ) ;
#46567=ADVANCED_FACE ( 'NONE', ( #32097 ), #55561, .F. ) ;
#46590=DIRECTION ( 'NONE',  ( -1.000000000000000000, -5.380183451256670742E-17, 1.298891185607911324E-16 ) ) ;
#46617=CARTESIAN_POINT ( 'NONE',  ( 42.00000000000000711, 0.000000000000000000, 0.000000000000000000 ) ) ;
#46684=FACE_OUTER_BOUND ( 'NONE', #60235, .T. ) ;
#46722=ORIENTED_EDGE ( 'NONE', *, *, #9009, .F. ) ;
#46933=DIRECTION ( 'NONE',  ( 1.000000000000000000, 1.558861125776144859E-16, -3.851859888774471706E-32 ) ) ;
#47006=ORIENTED_EDGE ( 'NONE', *, *, #59864, .F. ) ;
#47046=ORIENTED_EDGE ( 'NONE', *, *, #6161, .F. ) ;
#47141=CARTESIAN_POINT ( 'NONE',  ( 42.00000000000000711, 6.547216728259810428E-15, -1.617781153285278467E-30 ) ) ;
#47189=ORIENTED_EDGE ( 'NONE', *, *, #52505, .F. ) ;
#47203=LINE ( 'NONE', #23084, #33466 ) ;
#47241=ORIENTED_EDGE ( 'NONE', *, *, #22745, .T. ) ;
#47270=VERTEX_POINT ( 'NONE', #58157 ) ;
#47281=DIRECTION ( 'NONE',  ( -1.000000000000000000, -0.000000000000000000, -0.000000000000000000 ) ) ;
#47291=( NAMED_UNIT ( * ) SI_UNIT ( $, .STERADIAN. ) SOLID_ANGLE_UNIT ( ) );
#47344=EDGE_CURVE ( 'NONE', #12652, #24696, #10571, .T. ) ;
#47374=ADVANCED_FACE ( 'NONE', ( #59507 ), #8132, .F. ) ;
#47400=VERTEX_POINT ( 'NONE', #12862 ) ;
#47412=ORIENTED_EDGE ( 'NONE', *, *, #61718, .T. ) ;
#47448=DIRECTION ( 'NONE',  ( -1.000000000000000000, -5.380183451256670742E-17, 1.298891185607911324E-16 ) ) ;
#47472=FACE_OUTER_BOUND ( 'NONE', #5915, .T. ) ;
#47540=ORIENTED_EDGE ( 'NONE', *, *, #53884, .T. ) ;
#47545=DIRECTION ( 'NONE',  ( 1.000000000000000000, 1.836909530733573776E-16, -1.925929944387235579E-32 ) ) ;
#47636=ORIENTED_EDGE ( 'NONE', *, *, #27510, .F. ) ;
#47684=DIRECTION ( 'NONE',  ( 0.000000000000000000, -0.7071067811865435759, -0.7071067811865514585 ) ) ;
#47711=FACE_OUTER_BOUND ( 'NONE', #2625, .T. ) ;
#47761=DIRECTION ( 'NONE',  ( -1.000000000000000000, -1.836909530733580185E-16, 1.836909530733574022E-16 ) ) ;
#47810=EDGE_CURVE ( 'NONE', #58502, #51012, #60784, .T. ) ;
#47845=FACE_OUTER_BOUND ( 'NONE', #30155, .T. ) ;
#47911=AXIS2_PLACEMENT_3D ( 'NONE', #23637, #51820, #52747 ) ;
#47938=ORIENTED_EDGE ( 'NONE', *, *, #4020, .F. ) ;
#47940=CARTESIAN_POINT ( 'NONE',  ( 7.000000000000007105, -2.650000000000270806, 80.00000000000000000 ) ) ;
#47994=AXIS2_PLACEMENT_3D ( 'NONE', #12106, #40006, #30870 ) ;
#48027=CLOSED_SHELL ( 'NONE', ( #16345, #50524, #30267, #24660, #45225, #53805, #24460, #20348, #27226, #11884, #16073, #58467, #15641, #24045, #37080, #2034, #1308, #35324, #9709, #3408, #41234, #56482, #58599, #23788, #36878, #57608, #47374, #16635, #5227, #4221, #46567, #31465, #45413, #29416 ) ) ;
#48064=DIRECTION ( 'NONE',  ( -1.000000000000000000, -1.836909530733573529E-16, 1.361838123766461297E-32 ) ) ;
#48139=CARTESIAN_POINT ( 'NONE',  ( 42.00000000000000711, 7.805869035311033600E-47, 13.00000000000000178 ) ) ;
#48167=CIRCLE ( 'NONE', #61101, 2.649999999999992806 ) ;
#48180=CARTESIAN_POINT ( 'NONE',  ( 9.999999999999994671, 54.69470952478017978, -58.44237546506749226 ) ) ;
#48191=ORIENTED_EDGE ( 'NONE', *, *, #12076, .F. ) ;
#48208=CYLINDRICAL_SURFACE ( 'NONE', #4472, 13.00000000000000178 ) ;
#48235=ORIENTED_EDGE ( 'NONE', *, *, #8973, .T. ) ;
#48249=CIRCLE ( 'NONE', #33233, 2.649999999999997691 ) ;
#48250=ORIENTED_EDGE ( 'NONE', *, *, #732, .T. ) ;
#48339=CIRCLE ( 'NONE', #20358, 2.649999999999997691 ) ;
#48451=FACE_BOUND ( 'NONE', #16341, .T. ) ;
#48465=CIRCLE ( 'NONE', #43489, 2.649999999999992806 ) ;
#48534=DIRECTION ( 'NONE',  ( -1.000000000000000000, -0.000000000000000000, 1.925929944387235853E-32 ) ) ;
#48554=PLANE ( 'NONE',  #27094 ) ;
#48647=EDGE_CURVE ( 'NONE', #53393, #39665, #2739, .T. ) ;
#48656=DIRECTION ( 'NONE',  ( 0.000000000000000000, 0.000000000000000000, 1.000000000000000000 ) ) ;
#48690=DIRECTION ( 'NONE',  ( 1.000000000000000000, 1.836909530733573776E-16, -1.925929944387235579E-32 ) ) ;
#48840=STYLED_ITEM ( 'NONE', ( #14408 ), #4831 ) ;
#48931=EDGE_CURVE ( 'NONE', #50728, #55180, #13872, .T. ) ;
#48946=AXIS2_PLACEMENT_3D ( 'NONE', #60698, #21586, #26584 ) ;
#49007=VERTEX_POINT ( 'NONE', #59680 ) ;
#49112=ORIENTED_EDGE ( 'NONE', *, *, #20722, .T. ) ;
#49120=EDGE_LOOP ( 'NONE', ( #29659, #11785 ) ) ;
#49159=CARTESIAN_POINT ( 'NONE',  ( 10.00000000000000888, 0.000000000000000000, 0.000000000000000000 ) ) ;
#49302=DIRECTION ( 'NONE',  ( 0.000000000000000000, 0.000000000000000000, 1.000000000000000000 ) ) ;
#49343=DIRECTION ( 'NONE',  ( 1.850371707708593823E-16, -1.000000000000000000, 0.000000000000000000 ) ) ;
#49366=DIRECTION ( 'NONE',  ( 0.000000000000000000, 1.000000000000000000, 0.000000000000000000 ) ) ;
#49531=VERTEX_POINT ( 'NONE', #36305 ) ;
#49569=EDGE_CURVE ( 'NONE', #3017, #1874, #28825, .T. ) ;
#49657=CARTESIAN_POINT ( 'NONE',  ( 7.000000000000006217, 8.392413579938656024E-13, -80.00000000000001421 ) ) ;
#49891=DIRECTION ( 'NONE',  ( -1.000000000000000000, -1.836909530733554547E-16, -1.836909530733573529E-16 ) ) ;
#49907=CIRCLE ( 'NONE', #47911, 75.00000000000001421 ) ;
#49986=DIRECTION ( 'NONE',  ( 0.000000000000000000, 0.7071067811865382469, 0.7071067811865566766 ) ) ;
#50005=CARTESIAN_POINT ( 'NONE',  ( 45.00000000000001421, 1.592040838891559293E-15, -13.00000000000000178 ) ) ;
#50174=VERTEX_POINT ( 'NONE', #10170 ) ;
#50177=EDGE_LOOP ( 'NONE', ( #28074, #37514 ) ) ;
#50491=EDGE_CURVE ( 'NONE', #42003, #51041, #48339, .T. ) ;
#50524=ADVANCED_FACE ( 'NONE', ( #53848 ), #10352, .F. ) ;
#50570=( NAMED_UNIT ( * ) SI_UNIT ( $, .STERADIAN. ) SOLID_ANGLE_UNIT ( ) );
#50573=DIRECTION ( 'NONE',  ( -1.000000000000000000, -1.836909530733573776E-16, 1.925929944387235579E-32 ) ) ;
#50591=SHAPE_DEFINITION_REPRESENTATION ( #45814, #6760 ) ;
#50679=AXIS2_PLACEMENT_3D ( 'NONE', #21460, #50573, #6709 ) ;
#50728=VERTEX_POINT ( 'NONE', #18763 ) ;
#50847=( GEOMETRIC_REPRESENTATION_CONTEXT ( 3 ) GLOBAL_UNCERTAINTY_ASSIGNED_CONTEXT ( ( #51151 ) ) GLOBAL_UNIT_ASSIGNED_CONTEXT ( ( #53813, #11882, #11558 ) ) REPRESENTATION_CONTEXT ( 'NONE', 'WORKASPACE' ) );
#50864=AXIS2_PLACEMENT_3D ( 'NONE', #59040, #44076, #49343 ) ;
#50923=DIRECTION ( 'NONE',  ( 3.273063162220399693E-16, -1.000000000000000000, -5.236901059552639509E-15 ) ) ;
#50943=DIRECTION ( 'NONE',  ( 1.000000000000000000, 1.836909530733573776E-16, -1.925929944387235579E-32 ) ) ;
#50953=CARTESIAN_POINT ( 'NONE',  ( 6.999999999999995559, 56.56854249492450037, -56.56854249492312192 ) ) ;
#51012=VERTEX_POINT ( 'NONE', #25916 ) ;
#51041=VERTEX_POINT ( 'NONE', #3620 ) ;
#51063=LINE ( 'NONE', #27272, #52246 ) ;
#51151=UNCERTAINTY_MEASURE_WITH_UNIT (LENGTH_MEASURE( 1.000000000000000082E-05 ), #53813, 'distance_accuracy_value', 'NONE');
#51302=CARTESIAN_POINT ( 'NONE',  ( 30.00000000000001066, 4.342925291379521108E-15, -1.386669559958810165E-30 ) ) ;
#51396=CARTESIAN_POINT ( 'NONE',  ( 42.00000000000000711, 0.000000000000000000, 0.000000000000000000 ) ) ;
#51429=DIRECTION ( 'NONE',  ( -1.000000000000000000, -0.000000000000000000, 1.925929944387235853E-32 ) ) ;
#51536=CIRCLE ( 'NONE', #4529, 15.99999999999999645 ) ;
#51698=CARTESIAN_POINT ( 'NONE',  ( 9.999999999999994671, 56.56854249492450037, -56.56854249492312192 ) ) ;
#51775=CARTESIAN_POINT ( 'NONE',  ( 7.000000000000006217, 1.285836671513502038E-15, -1.348150961071066192E-31 ) ) ;
#51820=DIRECTION ( 'NONE',  ( 1.000000000000000000, 1.558861125776144859E-16, -3.851859888774471706E-32 ) ) ;
#51832=EDGE_LOOP ( 'NONE', ( #36103, #47189, #40334, #34918 ) ) ;
#51993=AXIS2_PLACEMENT_3D ( 'NONE', #46378, #23175, #22867 ) ;
#52011=ORIENTED_EDGE ( 'NONE', *, *, #36242, .F. ) ;
#52051=EDGE_CURVE ( 'NONE', #18005, #3387, #47203, .T. ) ;
#52219=CARTESIAN_POINT ( 'NONE',  ( 30.00000000000001066, 4.342925291379521108E-15, -1.386669559958810165E-30 ) ) ;
#52226=CYLINDRICAL_SURFACE ( 'NONE', #17222, 18.99999999999999645 ) ;
#52245=MANIFOLD_SOLID_BREP ( 'CirPattern1', #48027 ) ;
#52246=VECTOR ( 'NONE', #31983, 1000.000000000000000 ) ;
#52312=EDGE_LOOP ( 'NONE', ( #23136, #30618 ) ) ;
#52364=CARTESIAN_POINT ( 'NONE',  ( 10.00000000000000533, -2.774815975767171530E-13, 80.00000000000001421 ) ) ;
#52384=LINE ( 'NONE', #9171, #28930 ) ;
#52505=EDGE_CURVE ( 'NONE', #9955, #33012, #13428, .T. ) ;
#52575=VECTOR ( 'NONE', #3488, 1000.000000000000000 ) ;
#52627=CARTESIAN_POINT ( 'NONE',  ( 10.00000000000001599, -54.69470952477976766, 58.44237546506786884 ) ) ;
#52640=ORIENTED_EDGE ( 'NONE', *, *, #21700, .T. ) ;
#52747=DIRECTION ( 'NONE',  ( -1.850371707708593823E-16, 1.000000000000000000, 0.000000000000000000 ) ) ;
#52832=DIRECTION ( 'NONE',  ( -1.000000000000000000, -1.836909530733573776E-16, 2.465190328815655050E-32 ) ) ;
#52896=ORIENTED_EDGE ( 'NONE', *, *, #18393, .F. ) ;
#52929=DIRECTION ( 'NONE',  ( -1.000000000000000000, -1.836909530733580185E-16, 1.836909530733574022E-16 ) ) ;
#53090=EDGE_LOOP ( 'NONE', ( #18051, #56247 ) ) ;
#53195=AXIS2_PLACEMENT_3D ( 'NONE', #12744, #42187, #50923 ) ;
#53225=CARTESIAN_POINT ( 'NONE',  ( 6.999999999999991118, 80.00000000000001421, -7.414830285890871171E-32 ) ) ;
#53247=DIRECTION ( 'NONE',  ( -1.000000000000000000, -1.836909530733573776E-16, 1.925929944387235853E-32 ) ) ;
#53393=VERTEX_POINT ( 'NONE', #52627 ) ;
#53447=PLANE ( 'NONE',  #30471 ) ;
#53465=CARTESIAN_POINT ( 'NONE',  ( 7.000000000000006217, 8.392413579938656024E-13, -80.00000000000001421 ) ) ;
#53614=EDGE_CURVE ( 'NONE', #53393, #43245, #48465, .T. ) ;
#53805=ADVANCED_FACE ( 'NONE', ( #16209 ), #34398, .F. ) ;
#53813=( LENGTH_UNIT ( ) NAMED_UNIT ( * ) SI_UNIT ( .MILLI., .METRE. ) );
#53835=DIRECTION ( 'NONE',  ( -1.000000000000000000, -1.836909530733573776E-16, 1.925929944387235853E-32 ) ) ;
#53848=FACE_OUTER_BOUND ( 'NONE', #23461, .T. ) ;
#53870=ORIENTED_EDGE ( 'NONE', *, *, #732, .F. ) ;
#53884=EDGE_CURVE ( 'NONE', #43795, #4007, #46270, .T. ) ;
#53930=EDGE_CURVE ( 'NONE', #43245, #57549, #55014, .T. ) ;
#53981=VECTOR ( 'NONE', #30358, 1000.000000000000000 ) ;
#54048=DIRECTION ( 'NONE',  ( 1.000000000000000000, 1.558861125776144859E-16, -3.851859888774471706E-32 ) ) ;
#54075=CARTESIAN_POINT ( 'NONE',  ( 7.000000000000016875, -56.56854249492410958, 56.56854249492351983 ) ) ;
#54080=ORIENTED_EDGE ( 'NONE', *, *, #22639, .T. ) ;
#54086=ORIENTED_EDGE ( 'NONE', *, *, #37010, .T. ) ;
#54156=CARTESIAN_POINT ( 'NONE',  ( 7.000000000000016875, -56.56854249492410958, 56.56854249492351983 ) ) ;
#54215=EDGE_LOOP ( 'NONE', ( #38063, #20392 ) ) ;
#54282=FACE_BOUND ( 'NONE', #57777, .T. ) ;
#54285=CARTESIAN_POINT ( 'NONE',  ( 30.00000000000001421, -15.99999999999999289, 1.959434878635763159E-15 ) ) ;
#54311=CARTESIAN_POINT ( 'NONE',  ( 7.000000000000006217, 1.285836671513502038E-15, -1.348150961071066192E-31 ) ) ;
#54325=FILL_AREA_STYLE ('',( #60267 ) ) ;
#54392=STYLED_ITEM ( 'NONE', ( #12385 ), #52245 ) ;
#54408=CARTESIAN_POINT ( 'NONE',  ( 9.999999999999991118, 80.00000000000001421, -1.319262011905257654E-31 ) ) ;
#54432=AXIS2_PLACEMENT_3D ( 'NONE', #8262, #4173, #27383 ) ;
#54480=AXIS2_PLACEMENT_3D ( 'NONE', #6151, #21518, #16514 ) ;
#54600=CARTESIAN_POINT ( 'NONE',  ( 45.00000000000001421, 0.000000000000000000, 13.00000000000000178 ) ) ;
#54601=DIRECTION ( 'NONE',  ( -1.000000000000000000, -0.000000000000000000, -0.000000000000000000 ) ) ;
#54648=EDGE_CURVE ( 'NONE', #10608, #1988, #36551, .T. ) ;
#54743=CARTESIAN_POINT ( 'NONE',  ( 6.999999999999990230, 85.00000000000001421, 1.040949779275250495E-14 ) ) ;
#54750=CARTESIAN_POINT ( 'NONE',  ( 7.000000000000006217, 1.285836671513502826E-15, -1.348150961071066192E-31 ) ) ;
#54751=AXIS2_PLACEMENT_3D ( 'NONE', #27698, #17683, #27381 ) ;
#54783=DIRECTION ( 'NONE',  ( -1.000000000000000000, -1.836909530733554547E-16, -1.836909530733573529E-16 ) ) ;
#54858=ORIENTED_EDGE ( 'NONE', *, *, #13335, .T. ) ;
#54969=AXIS2_PLACEMENT_3D ( 'NONE', #54075, #21826, #55314 ) ;
#55014=LINE ( 'NONE', #40969, #18520 ) ;
#55140=EDGE_CURVE ( 'NONE', #2711, #21079, #61496, .T. ) ;
#55155=AXIS2_PLACEMENT_3D ( 'NONE', #33799, #43509, #229 ) ;
#55180=VERTEX_POINT ( 'NONE', #14845 ) ;
#55220=FACE_BOUND ( 'NONE', #52312, .T. ) ;
#55226=LINE ( 'NONE', #54600, #24286 ) ;
#55261=SURFACE_SIDE_STYLE ('',( #11448 ) ) ;
#55272=DIRECTION ( 'NONE',  ( -1.000000000000000000, -1.836909530733554547E-16, -1.836909530733573529E-16 ) ) ;
#55314=DIRECTION ( 'NONE',  ( 0.000000000000000000, -0.7071067811865449082, -0.7071067811865500152 ) ) ;
#55338=EDGE_CURVE ( 'NONE', #55726, #33072, #20575, .T. ) ;
#55342=AXIS2_PLACEMENT_3D ( 'NONE', #54156, #5607, #20679 ) ;
#55343=EDGE_CURVE ( 'NONE', #33072, #27868, #41444, .T. ) ;
#55372=EDGE_CURVE ( 'NONE', #9955, #10882, #22621, .T. ) ;
#55400=CARTESIAN_POINT ( 'NONE',  ( 10.00000000000002132, -80.00000000000001421, 2.649999999999992806 ) ) ;
#55402=VERTEX_POINT ( 'NONE', #32334 ) ;
#55517=VECTOR ( 'NONE', #23614, 1000.000000000000000 ) ;
#55552=ORIENTED_EDGE ( 'NONE', *, *, #23085, .F. ) ;
#55561=CYLINDRICAL_SURFACE ( 'NONE', #54751, 2.649999999999992806 ) ;
#55724=LINE ( 'NONE', #60730, #29766 ) ;
#55726=VERTEX_POINT ( 'NONE', #41674 ) ;
#55782=AXIS2_PLACEMENT_3D ( 'NONE', #45752, #11613, #35429 ) ;
#55912=FACE_OUTER_BOUND ( 'NONE', #42880, .T. ) ;
#56001=EDGE_CURVE ( 'NONE', #516, #27868, #51536, .T. ) ;
#56040=ORIENTED_EDGE ( 'NONE', *, *, #13183, .F. ) ;
#56149=ORIENTED_EDGE ( 'NONE', *, *, #16498, .F. ) ;
#56216=DIRECTION ( 'NONE',  ( 0.000000000000000000, 0.7071067811865527908, -0.7071067811865421326 ) ) ;
#56247=ORIENTED_EDGE ( 'NONE', *, *, #21933, .F. ) ;
#56295=DIRECTION ( 'NONE',  ( -1.000000000000000000, -1.836909530733580185E-16, 1.836909530733574022E-16 ) ) ;
#56320=CARTESIAN_POINT ( 'NONE',  ( 45.00000000000001421, 9.184850993605150311E-15, -75.00000000000001421 ) ) ;
#56348=CARTESIAN_POINT ( 'NONE',  ( 45.00000000000001421, 0.000000000000000000, 0.000000000000000000 ) ) ;
#56449=CIRCLE ( 'NONE', #2440, 2.649999999999999467 ) ;
#56482=ADVANCED_FACE ( 'NONE', ( #36295, #7123 ), #41610, .T. ) ;
#56607=CARTESIAN_POINT ( 'NONE',  ( 10.00000000000000888, 9.184850993605147156E-15, -75.00000000000001421 ) ) ;
#56745=CYLINDRICAL_SURFACE ( 'NONE', #25259, 2.649999999999997691 ) ;
#56789=AXIS2_PLACEMENT_3D ( 'NONE', #60301, #27120, #8009 ) ;
#56863=AXIS2_PLACEMENT_3D ( 'NONE', #9845, #48064, #61516 ) ;
#56897=DIRECTION ( 'NONE',  ( -1.000000000000000000, -1.836909530733573776E-16, 1.925929944387235579E-32 ) ) ;
#56923=DIRECTION ( 'NONE',  ( -1.000000000000000000, -1.836909530733573776E-16, 1.361838123766442686E-32 ) ) ;
#56969=CARTESIAN_POINT ( 'NONE',  ( 30.00000000000001066, 4.342925291379521108E-15, -1.386669559958810165E-30 ) ) ;
#57071=AXIS2_PLACEMENT_3D ( 'NONE', #32425, #17702, #32115 ) ;
#57073=ORIENTED_EDGE ( 'NONE', *, *, #53930, .T. ) ;
#57225=DIRECTION ( 'NONE',  ( -1.000000000000000000, -1.836909530733554547E-16, -1.836909530733573529E-16 ) ) ;
#57242=AXIS2_PLACEMENT_3D ( 'NONE', #60254, #17369, #27375 ) ;
#57274=SURFACE_STYLE_FILL_AREA ( #19717 ) ;
#57519=CYLINDRICAL_SURFACE ( 'NONE', #34776, 15.99999999999999645 ) ;
#57549=VERTEX_POINT ( 'NONE', #29346 ) ;
#57564=ORIENTED_EDGE ( 'NONE', *, *, #46280, .F. ) ;
#57608=ADVANCED_FACE ( 'NONE', ( #48451, #11178, #34999, #24656, #5519, #39089, #58143, #44707, #1747, #15268 ), #53447, .F. ) ;
#57777=EDGE_LOOP ( 'NONE', ( #56040, #11058 ) ) ;
#57840=FACE_OUTER_BOUND ( 'NONE', #30116, .T. ) ;
#57846=DIRECTION ( 'NONE',  ( -1.000000000000000000, -3.673819061467147552E-16, 1.925929944387234758E-32 ) ) ;
#57949=DIRECTION ( 'NONE',  ( 0.000000000000000000, -1.000000000000000000, 0.000000000000000000 ) ) ;
#58046=VECTOR ( 'NONE', #2684, 1000.000000000000000 ) ;
#58143=FACE_BOUND ( 'NONE', #9166, .T. ) ;
#58157=CARTESIAN_POINT ( 'NONE',  ( 10.00000000000000533, 2.649999999999715250, 80.00000000000002842 ) ) ;
#58209=SURFACE_STYLE_USAGE ( .BOTH. , #19114 ) ;
#58248=ORIENTED_EDGE ( 'NONE', *, *, #1045, .T. ) ;
#58306=DIRECTION ( 'NONE',  ( 0.000000000000000000, 1.000000000000000000, 0.000000000000000000 ) ) ;
#58434=CARTESIAN_POINT ( 'NONE',  ( 45.00000000000001421, 0.000000000000000000, 0.000000000000000000 ) ) ;
#58467=ADVANCED_FACE ( 'NONE', ( #37552 ), #60384, .F. ) ;
#58502=VERTEX_POINT ( 'NONE', #31912 ) ;
#58547=AXIS2_PLACEMENT_3D ( 'NONE', #17812, #34008, #36940 ) ;
#58549=ORIENTED_EDGE ( 'NONE', *, *, #27201, .T. ) ;
#58599=ADVANCED_FACE ( 'NONE', ( #26426 ), #7300, .T. ) ;
#58645=ORIENTED_EDGE ( 'NONE', *, *, #21700, .F. ) ;
#58772=CYLINDRICAL_SURFACE ( 'NONE', #54969, 2.649999999999992806 ) ;
#58943=CARTESIAN_POINT ( 'NONE',  ( 42.00000000000000711, 0.000000000000000000, 0.000000000000000000 ) ) ;
#59028=VERTEX_POINT ( 'NONE', #61088 ) ;
#59034=EDGE_CURVE ( 'NONE', #37250, #45271, #36547, .T. ) ;
#59035=DIRECTION ( 'NONE',  ( -1.000000000000000000, -1.836909530733573776E-16, -1.361838123766432833E-32 ) ) ;
#59040=CARTESIAN_POINT ( 'NONE',  ( 10.00000000000000888, 0.000000000000000000, 0.000000000000000000 ) ) ;
#59054=VECTOR ( 'NONE', #51429, 1000.000000000000000 ) ;
#59116=EDGE_CURVE ( 'NONE', #27605, #38027, #23818, .T. ) ;
#59140=CIRCLE ( 'NONE', #25118, 2.649999999999997691 ) ;
#59322=ORIENTED_EDGE ( 'NONE', *, *, #27201, .F. ) ;
#59427=CARTESIAN_POINT ( 'NONE',  ( 42.00000000000000711, 6.547216728259810428E-15, -1.617781153285278467E-30 ) ) ;
#59428=ORIENTED_EDGE ( 'NONE', *, *, #40316, .F. ) ;
#59507=FACE_OUTER_BOUND ( 'NONE', #7679, .T. ) ;
#59580=EDGE_LOOP ( 'NONE', ( #19995, #15011 ) ) ;
#59584=EDGE_CURVE ( 'NONE', #33012, #11927, #45038, .T. ) ;
#59616=DIRECTION ( 'NONE',  ( -1.000000000000000000, -1.836909530733573776E-16, 1.925929944387235853E-32 ) ) ;
#59630=VECTOR ( 'NONE', #23316, 1000.000000000000000 ) ;
#59634=EDGE_CURVE ( 'NONE', #21079, #45374, #3546, .T. ) ;
#59654=CARTESIAN_POINT ( 'NONE',  ( 10.00000000000001599, -56.56854249492331377, -56.56854249492430142 ) ) ;
#59665=DIRECTION ( 'NONE',  ( -1.000000000000000000, -1.836909530733580185E-16, 1.836909530733574022E-16 ) ) ;
#59680=CARTESIAN_POINT ( 'NONE',  ( 6.999999999999991118, 80.00000000000001421, -2.649999999999999467 ) ) ;
#59713=CARTESIAN_POINT ( 'NONE',  ( 41.99999999999999289, 72.00000000000004263, -4.718528363748728716E-31 ) ) ;
#59864=EDGE_CURVE ( 'NONE', #1874, #3017, #39635, .T. ) ;
#59883=DIRECTION ( 'NONE',  ( 1.836766033387207149E-16, -1.000000000000000000, 0.000000000000000000 ) ) ;
#59898=EDGE_CURVE ( 'NONE', #38431, #38620, #20613, .T. ) ;
#59902=ORIENTED_EDGE ( 'NONE', *, *, #46280, .T. ) ;
#59944=CARTESIAN_POINT ( 'NONE',  ( 30.00000000000001421, -18.99999999999999289, 2.326828918379968998E-15 ) ) ;
#59948=CARTESIAN_POINT ( 'NONE',  ( 30.00000000000001066, 4.342925291379521108E-15, -1.386669559958810165E-30 ) ) ;
#59968=DIRECTION ( 'NONE',  ( -1.000000000000000000, -0.000000000000000000, 1.925929944387235853E-32 ) ) ;
#59991=DIRECTION ( 'NONE',  ( -1.000000000000000000, -5.380183451256491399E-17, -1.298891185607892835E-16 ) ) ;
#60010=LINE ( 'NONE', #50005, #58046 ) ;
#60235=EDGE_LOOP ( 'NONE', ( #14542, #31441, #5603, #24601 ) ) ;
#60254=CARTESIAN_POINT ( 'NONE',  ( 45.00000000000001421, 0.000000000000000000, 0.000000000000000000 ) ) ;
#60267=FILL_AREA_STYLE_COLOUR ( '', #11411 ) ;
#60301=CARTESIAN_POINT ( 'NONE',  ( 10.00000000000000533, 8.397924308530857731E-13, -80.00000000000001421 ) ) ;
#60331=EDGE_LOOP ( 'NONE', ( #33857, #16082, #44751, #44273 ) ) ;
#60384=CYLINDRICAL_SURFACE ( 'NONE', #58547, 72.00000000000002842 ) ;
#60403=CARTESIAN_POINT ( 'NONE',  ( 7.000000000000016875, -58.44237546506768410, -54.69470952477996661 ) ) ;
#60666=CARTESIAN_POINT ( 'NONE',  ( 7.000000000000016875, -56.56854249492410958, 56.56854249492351983 ) ) ;
#60676=CARTESIAN_POINT ( 'NONE',  ( 30.00000000000001066, 4.342925291379521108E-15, -1.386669559958810165E-30 ) ) ;
#60698=CARTESIAN_POINT ( 'NONE',  ( 6.999999999999995559, 56.56854249492450037, -56.56854249492312192 ) ) ;
#60704=DIRECTION ( 'NONE',  ( -1.000000000000000000, -0.000000000000000000, -0.000000000000000000 ) ) ;
#60730=CARTESIAN_POINT ( 'NONE',  ( 10.00000000000002132, -85.00000000000001421, -1.925929944387237167E-31 ) ) ;
#60784=CIRCLE ( 'NONE', #34793, 18.99999999999999645 ) ;
#60867=EDGE_CURVE ( 'NONE', #2711, #18038, #44688, .T. ) ;
#60961=LINE ( 'NONE', #3624, #1982 ) ;
#61088=CARTESIAN_POINT ( 'NONE',  ( 9.999999999999991118, 80.00000000000001421, -2.649999999999992806 ) ) ;
#61095=CARTESIAN_POINT ( 'NONE',  ( 10.00000000000002132, -80.00000000000001421, -2.649999999999992806 ) ) ;
#61101=AXIS2_PLACEMENT_3D ( 'NONE', #6576, #25722, #12572 ) ;
#61387=DIRECTION ( 'NONE',  ( 0.000000000000000000, 0.000000000000000000, 1.000000000000000000 ) ) ;
#61496=LINE ( 'NONE', #37748, #55517 ) ;
#61516=DIRECTION ( 'NONE',  ( 0.000000000000000000, -0.7071067811865553443, 0.7071067811865395791 ) ) ;
#61534=LINE ( 'NONE', #54285, #45788 ) ;
#61546=AXIS2_PLACEMENT_3D ( 'NONE', #3848, #32698, #18914 ) ;
#61604=VECTOR ( 'NONE', #29945, 1000.000000000000000 ) ;
#61718=EDGE_CURVE ( 'NONE', #1357, #47400, #9693, .T. ) ;
#61821=FACE_OUTER_BOUND ( 'NONE', #18942, .T. ) ;
#61831=DIRECTION ( 'NONE',  ( -1.000000000000000000, -1.836909530733573776E-16, 1.925929944387235579E-32 ) ) ;
#61844=ORIENTED_EDGE ( 'NONE', *, *, #59634, .T. ) ;
#61848=AXIS2_PLACEMENT_3D ( 'NONE', #7288, #59616, #27044 ) ;
#61930=CIRCLE ( 'NONE', #31969, 75.00000000000001421 ) ;
ENDSEC;
END-ISO-10303-21;
